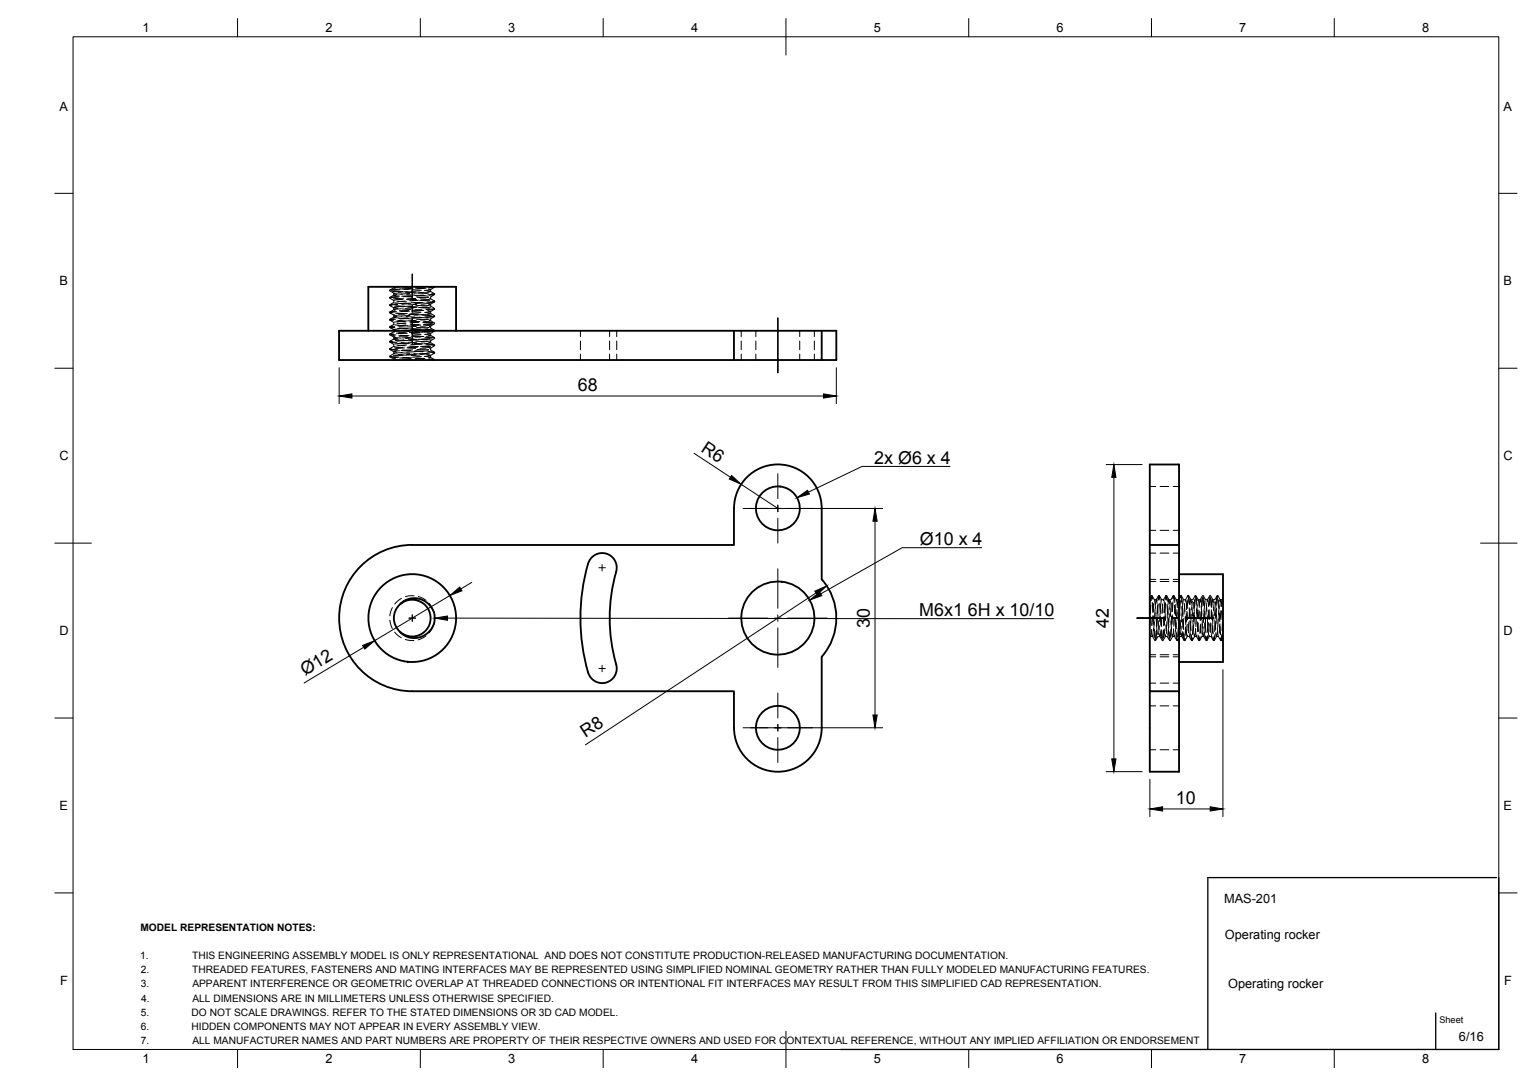
ISO-10303-21;
HEADER;
/* Generated by software containing ST-Developer
 * from STEP Tools, Inc. (www.steptools.com) 
 */

FILE_DESCRIPTION(
/* description */ ('Independent manual two-gate roller-track escapement for nominal30mm d
iameter20mm wide feed rollers. Opposed gates are driven by native capt
ured pin-slot loops with positive curved-slot travel stops at\X\B116de
g. Repeated gate/pin/washer/clip instances, adapted native common bear
ing families, full retaining lips and rotating polymer grip. External 
workpieces, gravity feeder/incline and mount anchors outside assembly.
 No powered-feed compatibility, impact, capacity, safety, force, wear 
or life rating.'),
/* implementation_level */ '2;1');

FILE_NAME(
/* name */ 'Operating rocker.step',
/* time_stamp */ '2026-11-08T18:43:23-08:00',
/* author */ (''),
/* organization */ (''),
/* preprocessor_version */ 'ST-DEVELOPER v20.2',
/* originating_system */ 'Autodesk Translation Framework v15.17.0.0',
/* authorisation */ '');

FILE_SCHEMA (('AUTOMOTIVE_DESIGN { 1 0 10303 214 3 1 1 }'));
ENDSEC;

DATA;
#10=MECHANICAL_DESIGN_GEOMETRIC_PRESENTATION_REPRESENTATION('',(#457),#19863);
#121=B_SPLINE_SURFACE_WITH_KNOTS('',3,3,((#14592,#14593,#14594,#14595,#14596,
#14597,#14598,#14599,#14600,#14601,#14602,#14603,#14604,#14605,#14606,#14607,
#14608,#14609,#14610,#14611,#14612,#14613,#14614,#14615,#14616,#14617,#14618,
#14619,#14620,#14621,#14622,#14623,#14624,#14625,#14626,#14627,#14628,#14629,
#14630,#14631,#14632,#14633,#14634,#14635,#14636,#14637,#14638,#14639,#14640,
#14641,#14642,#14643,#14644,#14645,#14646,#14647,#14648,#14649,#14650,#14651,
#14652,#14653,#14654,#14655,#14656,#14657,#14658,#14659),(#14660,#14661,
#14662,#14663,#14664,#14665,#14666,#14667,#14668,#14669,#14670,#14671,#14672,
#14673,#14674,#14675,#14676,#14677,#14678,#14679,#14680,#14681,#14682,#14683,
#14684,#14685,#14686,#14687,#14688,#14689,#14690,#14691,#14692,#14693,#14694,
#14695,#14696,#14697,#14698,#14699,#14700,#14701,#14702,#14703,#14704,#14705,
#14706,#14707,#14708,#14709,#14710,#14711,#14712,#14713,#14714,#14715,#14716,
#14717,#14718,#14719,#14720,#14721,#14722,#14723,#14724,#14725,#14726,#14727),
(#14728,#14729,#14730,#14731,#14732,#14733,#14734,#14735,#14736,#14737,
#14738,#14739,#14740,#14741,#14742,#14743,#14744,#14745,#14746,#14747,#14748,
#14749,#14750,#14751,#14752,#14753,#14754,#14755,#14756,#14757,#14758,#14759,
#14760,#14761,#14762,#14763,#14764,#14765,#14766,#14767,#14768,#14769,#14770,
#14771,#14772,#14773,#14774,#14775,#14776,#14777,#14778,#14779,#14780,#14781,
#14782,#14783,#14784,#14785,#14786,#14787,#14788,#14789,#14790,#14791,#14792,
#14793,#14794,#14795),(#14796,#14797,#14798,#14799,#14800,#14801,#14802,
#14803,#14804,#14805,#14806,#14807,#14808,#14809,#14810,#14811,#14812,#14813,
#14814,#14815,#14816,#14817,#14818,#14819,#14820,#14821,#14822,#14823,#14824,
#14825,#14826,#14827,#14828,#14829,#14830,#14831,#14832,#14833,#14834,#14835,
#14836,#14837,#14838,#14839,#14840,#14841,#14842,#14843,#14844,#14845,#14846,
#14847,#14848,#14849,#14850,#14851,#14852,#14853,#14854,#14855,#14856,#14857,
#14858,#14859,#14860,#14861,#14862,#14863)),.UNSPECIFIED.,.F.,.F.,.F.,(4,
4),(4,1,1,1,1,1,1,1,1,1,1,1,1,1,1,1,1,1,1,1,1,1,1,1,1,1,1,1,1,1,1,1,1,1,
1,1,1,1,1,1,1,1,1,1,1,1,1,1,1,1,1,1,1,1,1,1,1,1,1,1,1,1,1,1,1,4),(0.,0.0642013499338864),
(11.8589888623078,12.8566626771512,13.8543364919947,14.8520103068381,15.8496841216816,
16.8473579365251,17.8450317513685,18.842705566212,19.8403793810554,20.8380531958989,
21.8357270107423,22.8334008255858,23.8310746404292,24.8287484552727,25.8264222701161,
26.8240960849596,27.821769899803,28.8194437146465,29.8171175294899,30.8147913443334,
31.8124651591768,32.8101389740203,33.8078127888637,34.8054866037072,35.8031604185506,
36.8008342333941,37.7985080482375,38.796181863081,39.7938556779244,40.7915294927679,
41.7892033076113,42.7868771224548,43.7845509372982,44.7822247521417,45.7798985669851,
46.7775723818286,47.775246196672,48.7729200115155,49.7705938263589,50.7682676412024,
51.7659414560458,52.7636152708893,53.7612890857327,54.7589629005762,55.7566367154196,
56.7543105302631,57.7519843451065,58.74965815995,59.7473319747934,60.7450057896369,
61.7426796044803,62.7403534193238,63.7380272341672,64.7357010490107,65.7333748638542,
66.7310486786976,67.728722493541,68.7263963083845,69.7240701232279,70.7217439380714,
71.7194177529149,72.7170915677583,73.7147653826018,74.7124391974452,75.7101130122887,
76.7077868271321),.UNSPECIFIED.);
#122=B_SPLINE_SURFACE_WITH_KNOTS('',3,3,((#15080,#15081,#15082,#15083,#15084,
#15085,#15086,#15087,#15088,#15089,#15090,#15091,#15092,#15093,#15094,#15095,
#15096,#15097,#15098,#15099,#15100,#15101,#15102,#15103,#15104,#15105,#15106,
#15107,#15108,#15109,#15110,#15111,#15112,#15113,#15114,#15115,#15116,#15117,
#15118,#15119,#15120,#15121,#15122,#15123,#15124,#15125,#15126,#15127,#15128,
#15129,#15130,#15131,#15132,#15133,#15134,#15135,#15136,#15137,#15138,#15139,
#15140,#15141,#15142,#15143,#15144,#15145,#15146,#15147),(#15148,#15149,
#15150,#15151,#15152,#15153,#15154,#15155,#15156,#15157,#15158,#15159,#15160,
#15161,#15162,#15163,#15164,#15165,#15166,#15167,#15168,#15169,#15170,#15171,
#15172,#15173,#15174,#15175,#15176,#15177,#15178,#15179,#15180,#15181,#15182,
#15183,#15184,#15185,#15186,#15187,#15188,#15189,#15190,#15191,#15192,#15193,
#15194,#15195,#15196,#15197,#15198,#15199,#15200,#15201,#15202,#15203,#15204,
#15205,#15206,#15207,#15208,#15209,#15210,#15211,#15212,#15213,#15214,#15215),
(#15216,#15217,#15218,#15219,#15220,#15221,#15222,#15223,#15224,#15225,
#15226,#15227,#15228,#15229,#15230,#15231,#15232,#15233,#15234,#15235,#15236,
#15237,#15238,#15239,#15240,#15241,#15242,#15243,#15244,#15245,#15246,#15247,
#15248,#15249,#15250,#15251,#15252,#15253,#15254,#15255,#15256,#15257,#15258,
#15259,#15260,#15261,#15262,#15263,#15264,#15265,#15266,#15267,#15268,#15269,
#15270,#15271,#15272,#15273,#15274,#15275,#15276,#15277,#15278,#15279,#15280,
#15281,#15282,#15283),(#15284,#15285,#15286,#15287,#15288,#15289,#15290,
#15291,#15292,#15293,#15294,#15295,#15296,#15297,#15298,#15299,#15300,#15301,
#15302,#15303,#15304,#15305,#15306,#15307,#15308,#15309,#15310,#15311,#15312,
#15313,#15314,#15315,#15316,#15317,#15318,#15319,#15320,#15321,#15322,#15323,
#15324,#15325,#15326,#15327,#15328,#15329,#15330,#15331,#15332,#15333,#15334,
#15335,#15336,#15337,#15338,#15339,#15340,#15341,#15342,#15343,#15344,#15345,
#15346,#15347,#15348,#15349,#15350,#15351)),.UNSPECIFIED.,.F.,.F.,.F.,(4,
4),(4,1,1,1,1,1,1,1,1,1,1,1,1,1,1,1,1,1,1,1,1,1,1,1,1,1,1,1,1,1,1,1,1,1,
1,1,1,1,1,1,1,1,1,1,1,1,1,1,1,1,1,1,1,1,1,1,1,1,1,1,1,1,1,1,1,4),(0.,0.0642013499338864),
(14.3984001269718,15.3960739418153,16.3937477566587,17.3914215715022,18.3890953863456,
19.3867692011891,20.3844430160325,21.382116830876,22.3797906457194,23.3774644605629,
24.3751382754063,25.3728120902498,26.3704859050932,27.3681597199367,28.3658335347801,
29.3635073496236,30.361181164467,31.3588549793105,32.3565287941539,33.3542026089974,
34.3518764238408,35.3495502386843,36.3472240535278,37.3448978683712,38.3425716832147,
39.3402454980581,40.3379193129016,41.335593127745,42.3332669425885,43.3309407574319,
44.3286145722754,45.3262883871188,46.3239622019623,47.3216360168057,48.3193098316492,
49.3169836464926,50.3146574613361,51.3123312761795,52.310005091023,53.3076789058664,
54.3053527207099,55.3030265355533,56.3007003503968,57.2983741652402,58.2960479800837,
59.2937217949271,60.2913956097706,61.289069424614,62.2867432394575,63.2844170543009,
64.2820908691444,65.2797646839878,66.2774384988313,67.2751123136747,68.2727861285182,
69.2704599433616,70.2681337582051,71.2658075730485,72.263481387892,73.2611552027354,
74.2588290175789,75.2565028324223,76.2541766472658,77.2518504621092,78.2495242769527,
79.2471980917962),.UNSPECIFIED.);
#269=B_SPLINE_CURVE_WITH_KNOTS('',3,(#13855,#13856,#13857,#13858),
 .UNSPECIFIED.,.F.,.F.,(4,4),(64.141416212773,64.8487979648243),
 .UNSPECIFIED.);
#270=B_SPLINE_CURVE_WITH_KNOTS('',3,(#13861,#13862,#13863,#13864,#13865,
#13866,#13867,#13868,#13869,#13870),.UNSPECIFIED.,.F.,.F.,(4,3,3,4),(-62.8318530717959,
-61.855776520294,-60.8581027054505,-60.3976421702574),.UNSPECIFIED.);
#271=B_SPLINE_CURVE_WITH_KNOTS('',3,(#13875,#13876,#13877,#13878,#13879,
#13880,#13881,#13882,#13883,#13884,#13885,#13886,#13887,#13888,#13889,#13890,
#13891,#13892,#13893,#13894,#13895,#13896,#13897,#13898,#13899),
 .UNSPECIFIED.,.F.,.F.,(4,3,3,3,3,3,3,3,4),(57.8582309055934,57.8650812609202,
58.8627550757636,59.8604288906071,60.8581027054505,61.855776520294,62.8534503351374,
63.8511241499809,64.141416212773),.UNSPECIFIED.);
#272=B_SPLINE_CURVE_WITH_KNOTS('',3,(#13900,#13901,#13902,#13903,#13904,
#13905,#13906,#13907,#13908,#13909,#13910,#13911,#13912,#13913,#13914,#13915,
#13916,#13917,#13918,#13919,#13920,#13921),.UNSPECIFIED.,.F.,.F.,(4,3,3,
3,3,3,3,4),(-60.3976421702574,-59.8604288906071,-58.8627550757636,-57.8650812609202,
-56.8674074460767,-55.8697336312333,-54.8720598163898,-54.1144568630778),
 .UNSPECIFIED.);
#273=B_SPLINE_CURVE_WITH_KNOTS('',3,(#13926,#13927,#13928,#13929,#13930,
#13931,#13932,#13933,#13934,#13935,#13936,#13937,#13938,#13939,#13940,#13941,
#13942,#13943,#13944,#13945,#13946,#13947),.UNSPECIFIED.,.F.,.F.,(4,3,3,
3,3,3,3,4),(51.5750455984138,51.8790383718595,52.8767121867029,53.8743860015464,
54.8720598163898,55.8697336312333,56.8674074460767,57.8582309055934),
 .UNSPECIFIED.);
#274=B_SPLINE_CURVE_WITH_KNOTS('',3,(#13948,#13949,#13950,#13951,#13952,
#13953,#13954,#13955,#13956,#13957,#13958,#13959,#13960,#13961,#13962,#13963,
#13964,#13965,#13966,#13967,#13968,#13969,#13970,#13971,#13972),
 .UNSPECIFIED.,.F.,.F.,(4,3,3,3,3,3,3,3,4),(-54.1144568630778,-53.8743860015464,
-52.8767121867029,-51.8790383718595,-50.881364557016,-49.8836907421725,
-48.8860169273291,-47.8883431124856,-47.8312715558982),.UNSPECIFIED.);
#275=B_SPLINE_CURVE_WITH_KNOTS('',3,(#13977,#13978,#13979,#13980,#13981,
#13982,#13983,#13984,#13985,#13986,#13987,#13988,#13989,#13990,#13991,#13992,
#13993,#13994,#13995,#13996,#13997,#13998),.UNSPECIFIED.,.F.,.F.,(4,3,3,
3,3,3,3,4),(45.2918602912342,45.8929954827987,46.8906692976422,47.8883431124856,
48.8860169273291,49.8836907421725,50.881364557016,51.5750455984138),
 .UNSPECIFIED.);
#276=B_SPLINE_CURVE_WITH_KNOTS('',3,(#13999,#14000,#14001,#14002,#14003,
#14004,#14005,#14006,#14007,#14008,#14009,#14010,#14011,#14012,#14013,#14014,
#14015,#14016,#14017,#14018,#14019,#14020),.UNSPECIFIED.,.F.,.F.,(4,3,3,
3,3,3,3,4),(-47.8312715558982,-46.8906692976422,-45.8929954827987,-44.8953216679553,
-43.8976478531118,-42.8999740382684,-41.9023002234249,-41.5480862487187),
 .UNSPECIFIED.);
#277=B_SPLINE_CURVE_WITH_KNOTS('',3,(#14025,#14026,#14027,#14028,#14029,
#14030,#14031,#14032,#14033,#14034,#14035,#14036,#14037,#14038,#14039,#14040,
#14041,#14042,#14043,#14044,#14045,#14046),.UNSPECIFIED.,.F.,.F.,(4,3,3,
3,3,3,3,4),(39.0086749840546,39.906952593738,40.9046264085815,41.9023002234249,
42.8999740382684,43.8976478531118,44.8953216679553,45.2918602912342),
 .UNSPECIFIED.);
#278=B_SPLINE_CURVE_WITH_KNOTS('',3,(#14047,#14048,#14049,#14050,#14051,
#14052,#14053,#14054,#14055,#14056,#14057,#14058,#14059,#14060,#14061,#14062,
#14063,#14064,#14065,#14066,#14067,#14068),.UNSPECIFIED.,.F.,.F.,(4,3,3,
3,3,3,3,4),(-41.5480862487187,-40.9046264085815,-39.906952593738,-38.9092787788946,
-37.9116049640511,-36.9139311492077,-35.9162573343642,-35.2649009415391),
 .UNSPECIFIED.);
#279=B_SPLINE_CURVE_WITH_KNOTS('',3,(#14073,#14074,#14075,#14076,#14077,
#14078,#14079,#14080,#14081,#14082,#14083,#14084,#14085,#14086,#14087,#14088,
#14089,#14090,#14091,#14092,#14093,#14094,#14095,#14096,#14097),
 .UNSPECIFIED.,.F.,.F.,(4,3,3,3,3,3,3,3,4),(32.725489676875,32.9232358898339,
33.9209097046773,34.9185835195208,35.9162573343642,36.9139311492077,37.9116049640511,
38.9092787788946,39.0086749840546),.UNSPECIFIED.);
#280=B_SPLINE_CURVE_WITH_KNOTS('',3,(#14098,#14099,#14100,#14101,#14102,
#14103,#14104,#14105,#14106,#14107,#14108,#14109,#14110,#14111,#14112,#14113,
#14114,#14115,#14116,#14117,#14118,#14119),.UNSPECIFIED.,.F.,.F.,(4,3,3,
3,3,3,3,4),(-35.2649009415391,-34.9185835195208,-33.9209097046773,-32.9232358898339,
-31.9255620749904,-30.927888260147,-29.9302144453035,-28.9817156343595),
 .UNSPECIFIED.);
#281=B_SPLINE_CURVE_WITH_KNOTS('',3,(#14124,#14125,#14126,#14127,#14128,
#14129,#14130,#14131,#14132,#14133,#14134,#14135,#14136,#14137,#14138,#14139,
#14140,#14141,#14142,#14143,#14144,#14145),.UNSPECIFIED.,.F.,.F.,(4,3,3,
3,3,3,3,4),(26.4423043696954,26.9371930007732,27.9348668156166,28.9325406304601,
29.9302144453035,30.927888260147,31.9255620749904,32.725489676875),
 .UNSPECIFIED.);
#282=B_SPLINE_CURVE_WITH_KNOTS('',3,(#14146,#14147,#14148,#14149,#14150,
#14151,#14152,#14153,#14154,#14155,#14156,#14157,#14158,#14159,#14160,#14161,
#14162,#14163,#14164,#14165,#14166,#14167,#14168,#14169,#14170),
 .UNSPECIFIED.,.F.,.F.,(4,3,3,3,3,3,3,3,4),(-28.9817156343595,-28.9325406304601,
-27.9348668156166,-26.9371930007732,-25.9395191859297,-24.9418453710863,
-23.9441715562428,-22.9464977413994,-22.6985303271799),.UNSPECIFIED.);
#283=B_SPLINE_CURVE_WITH_KNOTS('',3,(#14175,#14176,#14177,#14178,#14179,
#14180,#14181,#14182,#14183,#14184,#14185,#14186,#14187,#14188,#14189,#14190,
#14191,#14192,#14193,#14194,#14195,#14196),.UNSPECIFIED.,.F.,.F.,(4,3,3,
3,3,3,3,4),(20.1591190625158,20.9511501117125,21.9488239265559,22.9464977413994,
23.9441715562428,24.9418453710863,25.9395191859297,26.4423043696954),
 .UNSPECIFIED.);
#284=B_SPLINE_CURVE_WITH_KNOTS('',3,(#14197,#14198,#14199,#14200,#14201,
#14202,#14203,#14204,#14205,#14206,#14207,#14208,#14209,#14210,#14211,#14212,
#14213,#14214,#14215,#14216,#14217,#14218),.UNSPECIFIED.,.F.,.F.,(4,3,3,
3,3,3,3,4),(-22.6985303271799,-21.9488239265559,-20.9511501117125,-19.953476296869,
-18.9558024820256,-17.9581286671821,-16.9604548523387,-16.4153450200003),
 .UNSPECIFIED.);
#285=B_SPLINE_CURVE_WITH_KNOTS('',3,(#14223,#14224,#14225,#14226,#14227,
#14228,#14229,#14230,#14231,#14232,#14233,#14234,#14235,#14236,#14237,#14238,
#14239,#14240,#14241,#14242,#14243,#14244,#14245,#14246,#14247),
 .UNSPECIFIED.,.F.,.F.,(4,3,3,3,3,3,3,3,4),(13.8759337553362,13.9674334078083,
14.9651072226518,15.9627810374952,16.9604548523387,17.9581286671821,18.9558024820256,
19.953476296869,20.1591190625158),.UNSPECIFIED.);
#286=B_SPLINE_CURVE_WITH_KNOTS('',3,(#14248,#14249,#14250,#14251,#14252,
#14253,#14254,#14255,#14256,#14257,#14258,#14259,#14260,#14261,#14262,#14263,
#14264,#14265,#14266,#14267,#14268,#14269),.UNSPECIFIED.,.F.,.F.,(4,3,3,
3,3,3,3,4),(-16.4153450200003,-15.9627810374952,-14.9651072226518,-13.9674334078083,
-12.9697595929649,-11.9720857781214,-10.974411963278,-10.1321597128207),
 .UNSPECIFIED.);
#287=B_SPLINE_CURVE_WITH_KNOTS('',3,(#14275,#14276,#14277,#14278,#14279,
#14280,#14281,#14282,#14283,#14284,#14285,#14286,#14287),.UNSPECIFIED.,
 .F.,.F.,(4,3,3,3,4),(-3.84897440564113,-2.99302144453035,-1.9953476296869,
-0.997673814843452,0.),.UNSPECIFIED.);
#288=B_SPLINE_CURVE_WITH_KNOTS('',3,(#14290,#14291,#14292,#14293,#14294,
#14295,#14296,#14297,#14298,#14299,#14300,#14301,#14302,#14303,#14304,#14305,
#14306,#14307,#14308),.UNSPECIFIED.,.F.,.F.,(4,3,3,3,3,3,4),(2.01694489302847,
2.99302144453035,3.9906952593738,4.98836907421726,5.98604288906071,6.98371670390416,
7.59274844815664),.UNSPECIFIED.);
#289=B_SPLINE_CURVE_WITH_KNOTS('',3,(#14314,#14315,#14316,#14317,#14318,
#14319,#14320,#14321),.UNSPECIFIED.,.F.,.F.,(4,1,1,1,1,4),(72.2566310325652,
72.7170915677583,73.7147653826018,74.7124391974452,75.7101130122887,76.7077868271321),
 .UNSPECIFIED.);
#290=B_SPLINE_CURVE_WITH_KNOTS('',3,(#14324,#14325,#14326,#14327,#14328,
#14329,#14330,#14331,#14332),.UNSPECIFIED.,.F.,.F.,(4,1,1,1,1,1,4),(72.2566310325652,
72.263481387892,73.2611552027354,74.2588290175789,75.2565028324223,76.2541766472658,
77.2302531987677),.UNSPECIFIED.);
#291=B_SPLINE_CURVE_WITH_KNOTS('',3,(#14337,#14338,#14339,#14340,#14341,
#14342,#14343,#14344,#14345,#14346),.UNSPECIFIED.,.F.,.F.,(4,1,1,1,1,1,
1,4),(65.9734457253856,66.7310486786976,67.728722493541,68.7263963083845,
69.7240701232279,70.7217439380714,71.7194177529149,72.2566310325652),
 .UNSPECIFIED.);
#292=B_SPLINE_CURVE_WITH_KNOTS('',3,(#14347,#14348,#14349,#14350,#14351,
#14352,#14353,#14354,#14355,#14356),.UNSPECIFIED.,.F.,.F.,(4,1,1,1,1,1,
1,4),(65.9734457253856,66.2774384988313,67.2751123136747,68.2727861285182,
69.2704599433616,70.2681337582051,71.2658075730485,72.2566310325652),
 .UNSPECIFIED.);
#293=B_SPLINE_CURVE_WITH_KNOTS('',3,(#14361,#14362,#14363,#14364,#14365,
#14366,#14367,#14368,#14369,#14370,#14371),.UNSPECIFIED.,.F.,.F.,(4,1,1,
1,1,1,1,1,4),(59.6902604182061,59.7473319747934,60.7450057896369,61.7426796044803,
62.7403534193238,63.7380272341672,64.7357010490107,65.7333748638542,65.9734457253856),
 .UNSPECIFIED.);
#294=B_SPLINE_CURVE_WITH_KNOTS('',3,(#14372,#14373,#14374,#14375,#14376,
#14377,#14378,#14379,#14380,#14381),.UNSPECIFIED.,.F.,.F.,(4,1,1,1,1,1,
1,4),(59.6902604182061,60.2913956097706,61.289069424614,62.2867432394575,
63.2844170543009,64.2820908691444,65.2797646839878,65.9734457253856),
 .UNSPECIFIED.);
#295=B_SPLINE_CURVE_WITH_KNOTS('',3,(#14386,#14387,#14388,#14389,#14390,
#14391,#14392,#14393,#14394,#14395),.UNSPECIFIED.,.F.,.F.,(4,1,1,1,1,1,
1,4),(53.4070751110265,53.7612890857327,54.7589629005762,55.7566367154196,
56.7543105302631,57.7519843451065,58.74965815995,59.6902604182061),
 .UNSPECIFIED.);
#296=B_SPLINE_CURVE_WITH_KNOTS('',3,(#14396,#14397,#14398,#14399,#14400,
#14401,#14402,#14403,#14404,#14405),.UNSPECIFIED.,.F.,.F.,(4,1,1,1,1,1,
1,4),(53.4070751110265,54.3053527207099,55.3030265355533,56.3007003503968,
57.2983741652402,58.2960479800837,59.2937217949271,59.6902604182061),
 .UNSPECIFIED.);
#297=B_SPLINE_CURVE_WITH_KNOTS('',3,(#14410,#14411,#14412,#14413,#14414,
#14415,#14416,#14417,#14418,#14419),.UNSPECIFIED.,.F.,.F.,(4,1,1,1,1,1,
1,4),(47.1238898038469,47.775246196672,48.7729200115155,49.7705938263589,
50.7682676412024,51.7659414560458,52.7636152708893,53.4070751110265),
 .UNSPECIFIED.);
#298=B_SPLINE_CURVE_WITH_KNOTS('',3,(#14420,#14421,#14422,#14423,#14424,
#14425,#14426,#14427,#14428,#14429,#14430),.UNSPECIFIED.,.F.,.F.,(4,1,1,
1,1,1,1,1,4),(47.1238898038469,47.3216360168057,48.3193098316492,49.3169836464926,
50.3146574613361,51.3123312761795,52.310005091023,53.3076789058664,53.4070751110265),
 .UNSPECIFIED.);
#299=B_SPLINE_CURVE_WITH_KNOTS('',3,(#14435,#14436,#14437,#14438,#14439,
#14440,#14441,#14442,#14443,#14444),.UNSPECIFIED.,.F.,.F.,(4,1,1,1,1,1,
1,4),(40.8407044966673,41.7892033076113,42.7868771224548,43.7845509372982,
44.7822247521417,45.7798985669851,46.7775723818286,47.1238898038469),
 .UNSPECIFIED.);
#300=B_SPLINE_CURVE_WITH_KNOTS('',3,(#14445,#14446,#14447,#14448,#14449,
#14450,#14451,#14452,#14453,#14454),.UNSPECIFIED.,.F.,.F.,(4,1,1,1,1,1,
1,4),(40.8407044966673,41.335593127745,42.3332669425885,43.3309407574319,
44.3286145722754,45.3262883871188,46.3239622019623,47.1238898038469),
 .UNSPECIFIED.);
#301=B_SPLINE_CURVE_WITH_KNOTS('',3,(#14459,#14460,#14461,#14462,#14463,
#14464,#14465,#14466,#14467,#14468,#14469),.UNSPECIFIED.,.F.,.F.,(4,1,1,
1,1,1,1,1,4),(34.5575191894877,34.8054866037072,35.8031604185506,36.8008342333941,
37.7985080482375,38.796181863081,39.7938556779244,40.7915294927679,40.8407044966673),
 .UNSPECIFIED.);
#302=B_SPLINE_CURVE_WITH_KNOTS('',3,(#14470,#14471,#14472,#14473,#14474,
#14475,#14476,#14477,#14478,#14479),.UNSPECIFIED.,.F.,.F.,(4,1,1,1,1,1,
1,4),(34.5575191894877,35.3495502386843,36.3472240535278,37.3448978683712,
38.3425716832147,39.3402454980581,40.3379193129016,40.8407044966673),
 .UNSPECIFIED.);
#303=B_SPLINE_CURVE_WITH_KNOTS('',3,(#14484,#14485,#14486,#14487,#14488,
#14489,#14490,#14491,#14492,#14493),.UNSPECIFIED.,.F.,.F.,(4,1,1,1,1,1,
1,4),(28.2743338823081,28.8194437146465,29.8171175294899,30.8147913443334,
31.8124651591768,32.8101389740203,33.8078127888637,34.5575191894877),
 .UNSPECIFIED.);
#304=B_SPLINE_CURVE_WITH_KNOTS('',3,(#14494,#14495,#14496,#14497,#14498,
#14499,#14500,#14501,#14502,#14503,#14504),.UNSPECIFIED.,.F.,.F.,(4,1,1,
1,1,1,1,1,4),(28.2743338823081,28.3658335347801,29.3635073496236,30.361181164467,
31.3588549793105,32.3565287941539,33.3542026089974,34.3518764238408,34.5575191894877),
 .UNSPECIFIED.);
#305=B_SPLINE_CURVE_WITH_KNOTS('',3,(#14509,#14510,#14511,#14512,#14513,
#14514,#14515,#14516,#14517,#14518),.UNSPECIFIED.,.F.,.F.,(4,1,1,1,1,1,
1,4),(21.9911485751285,22.8334008255858,23.8310746404292,24.8287484552727,
25.8264222701161,26.8240960849596,27.821769899803,28.2743338823081),
 .UNSPECIFIED.);
#306=B_SPLINE_CURVE_WITH_KNOTS('',3,(#14519,#14520,#14521,#14522,#14523,
#14524,#14525,#14526,#14527,#14528),.UNSPECIFIED.,.F.,.F.,(4,1,1,1,1,1,
1,4),(21.9911485751285,22.3797906457194,23.3774644605629,24.3751382754063,
25.3728120902498,26.3704859050932,27.3681597199367,28.2743338823081),
 .UNSPECIFIED.);
#307=B_SPLINE_CURVE_WITH_KNOTS('',3,(#14534,#14535,#14536,#14537,#14538),
 .UNSPECIFIED.,.F.,.F.,(4,1,4),(14.3984001269718,15.3960739418153,15.7079632679489),
 .UNSPECIFIED.);
#308=B_SPLINE_CURVE_WITH_KNOTS('',3,(#14541,#14542,#14543,#14544,#14545),
 .UNSPECIFIED.,.F.,.F.,(4,1,4),(13.8759337553362,14.8520103068381,15.7079632679489),
 .UNSPECIFIED.);
#309=B_SPLINE_CURVE_WITH_KNOTS('',3,(#14571,#14572,#14573,#14574,#14575,
#14576,#14577,#14578,#14579,#14580,#14581),.UNSPECIFIED.,.F.,.F.,(4,1,1,
1,1,1,1,1,4),(15.7079632679489,15.8496841216816,16.8473579365251,17.8450317513685,
18.842705566212,19.8403793810554,20.8380531958989,21.8357270107423,21.9911485751285),
 .UNSPECIFIED.);
#310=B_SPLINE_CURVE_WITH_KNOTS('',3,(#14582,#14583,#14584,#14585,#14586,
#14587,#14588,#14589,#14590,#14591),.UNSPECIFIED.,.F.,.F.,(4,1,1,1,1,1,
1,4),(15.7079632679489,16.3937477566587,17.3914215715022,18.3890953863456,
19.3867692011891,20.3844430160325,21.382116830876,21.9911485751285),
 .UNSPECIFIED.);
#311=B_SPLINE_CURVE_WITH_KNOTS('',3,(#14864,#14865,#14866,#14867,#14868,
#14869,#14870,#14871,#14872,#14873,#14874,#14875,#14876,#14877,#14878,#14879,
#14880,#14881,#14882,#14883,#14884,#14885,#14886,#14887,#14888,#14889,#14890,
#14891,#14892,#14893,#14894,#14895,#14896,#14897,#14898,#14899,#14900,#14901,
#14902,#14903,#14904,#14905,#14906,#14907,#14908,#14909,#14910,#14911,#14912,
#14913,#14914,#14915,#14916,#14917,#14918,#14919,#14920,#14921,#14922,#14923,
#14924,#14925,#14926,#14927,#14928,#14929,#14930,#14931,#14932,#14933,#14934,
#14935,#14936,#14937,#14938,#14939,#14940,#14941,#14942,#14943,#14944,#14945,
#14946,#14947,#14948,#14949,#14950,#14951,#14952,#14953,#14954,#14955,#14956,
#14957),.UNSPECIFIED.,.F.,.F.,(4,3,3,3,3,3,3,3,3,3,3,3,3,3,3,3,3,3,3,3,
3,3,3,3,3,3,3,3,3,3,3,4),(0.,0.0297266436256191,0.060112679207304,0.0895302342422888,
0.115270594897901,0.120663503251604,0.150426428066333,0.180024192439473,
0.208881424201401,0.221328323689936,0.230189025923113,0.234057622905472,
0.262601272727233,0.290514012411483,0.295453119487182,0.324405121619328,
0.334115029800546,0.339546867385313,0.343311613769743,0.371402114253626,
0.399548690384148,0.427297276293485,0.438085418679347,0.44385539363774,
0.448937718500496,0.477641070286612,0.499168584126198,0.508042229411102,
0.513343363411791,0.539241448194656,0.563751125644958,0.56924861039943),
 .UNSPECIFIED.);
#312=B_SPLINE_CURVE_WITH_KNOTS('',3,(#14958,#14959,#14960,#14961,#14962,
#14963,#14964,#14965,#14966,#14967,#14968,#14969,#14970,#14971,#14972,#14973,
#14974,#14975,#14976,#14977,#14978,#14979,#14980,#14981,#14982,#14983,#14984,
#14985,#14986,#14987,#14988,#14989,#14990,#14991,#14992,#14993,#14994,#14995,
#14996,#14997,#14998,#14999,#15000,#15001,#15002,#15003,#15004,#15005,#15006,
#15007,#15008,#15009,#15010,#15011,#15012,#15013,#15014,#15015,#15016,#15017,
#15018,#15019,#15020,#15021,#15022,#15023,#15024,#15025,#15026,#15027,#15028,
#15029,#15030,#15031,#15032,#15033,#15034,#15035,#15036,#15037,#15038,#15039,
#15040,#15041,#15042,#15043,#15044,#15045,#15046,#15047,#15048,#15049,#15050,
#15051,#15052,#15053,#15054),.UNSPECIFIED.,.F.,.F.,(4,3,3,3,3,3,3,3,3,3,
3,3,3,3,3,3,3,3,3,3,3,3,3,3,3,3,3,3,3,3,3,3,4),(0.,0.0253663834374841,0.0514041120650232,
0.0783366031747472,0.0901195680352514,0.0965544176388419,0.102698656155734,
0.130005061278407,0.157761496023994,0.185037132253699,0.195822334387975,
0.20220621696723,0.20645540248052,0.235058614057351,0.263563013331617,0.266864040942815,
0.294770641765994,0.305810449331027,0.3111858125117,0.31568945545677,0.343780872272608,
0.372913770005713,0.40236688452419,0.41382997653101,0.422924087167126,0.42812442164653,
0.458189344870008,0.483694943608004,0.492094089615772,0.498168184514284,
0.529189962168139,0.560211739821994,0.566847306048124),.UNSPECIFIED.);
#313=B_SPLINE_CURVE_WITH_KNOTS('',3,(#15055,#15056,#15057,#15058,#15059,
#15060,#15061,#15062,#15063,#15064,#15065,#15066,#15067,#15068,#15069,#15070,
#15071,#15072,#15073,#15074,#15075,#15076,#15077,#15078,#15079),
 .UNSPECIFIED.,.F.,.F.,(4,3,3,3,3,3,3,3,4),(-10.1321597128207,-9.97673814843451,
-8.97906433359106,-7.98139051874761,-6.98371670390416,-5.9860428890607,
-4.98836907421726,-3.99069525937381,-3.84897440564113),.UNSPECIFIED.);
#314=B_SPLINE_CURVE_WITH_KNOTS('',3,(#15352,#15353,#15354,#15355,#15356,
#15357,#15358,#15359,#15360,#15361,#15362,#15363,#15364,#15365,#15366,#15367,
#15368,#15369,#15370,#15371,#15372,#15373,#15374,#15375,#15376,#15377,#15378,
#15379,#15380,#15381,#15382,#15383,#15384,#15385,#15386,#15387,#15388,#15389,
#15390,#15391,#15392,#15393,#15394,#15395,#15396,#15397,#15398,#15399,#15400,
#15401,#15402,#15403,#15404,#15405,#15406,#15407,#15408,#15409,#15410,#15411,
#15412,#15413,#15414,#15415,#15416,#15417,#15418,#15419,#15420,#15421,#15422,
#15423,#15424,#15425,#15426,#15427,#15428,#15429,#15430,#15431,#15432,#15433,
#15434,#15435,#15436,#15437,#15438,#15439,#15440,#15441,#15442,#15443,#15444,
#15445,#15446,#15447,#15448),.UNSPECIFIED.,.F.,.F.,(4,3,3,3,3,3,3,3,3,3,
3,3,3,3,3,3,3,3,3,3,3,3,3,3,3,3,3,3,3,3,3,3,4),(0.,0.0253664359602338,0.0514042119244802,
0.0783366905517712,0.0901196499512111,0.0965544540618819,0.102698644967743,
0.130005086208347,0.157761538287333,0.185037163951202,0.195822342994834,
0.20220622673851,0.206455408544716,0.235058628439391,0.26356301086795,0.266864040942809,
0.29477061610912,0.305810395174784,0.311185261381901,0.315689367741021,
0.343780744986089,0.372913624523944,0.402366734593413,0.413829681327142,
0.422920909218603,0.428124127377988,0.458189039903474,0.483694714883097,
0.492093067075374,0.498168205826972,0.529189972824469,0.560211739821966,
0.566847306048091),.UNSPECIFIED.);
#315=B_SPLINE_CURVE_WITH_KNOTS('',3,(#15449,#15450,#15451,#15452,#15453,
#15454,#15455,#15456,#15457,#15458,#15459,#15460,#15461,#15462,#15463,#15464,
#15465,#15466,#15467,#15468,#15469,#15470),.UNSPECIFIED.,.F.,.F.,(4,3,3,
3,3,3,3,4),(7.59274844815664,7.98139051874761,8.97906433359106,9.97673814843451,
10.974411963278,11.9720857781214,12.9697595929649,13.8759337553362),
 .UNSPECIFIED.);
#316=B_SPLINE_CURVE_WITH_KNOTS('',3,(#15471,#15472,#15473,#15474,#15475,
#15476,#15477,#15478,#15479,#15480,#15481,#15482,#15483,#15484,#15485,#15486,
#15487,#15488,#15489,#15490,#15491,#15492,#15493,#15494,#15495,#15496,#15497,
#15498,#15499,#15500,#15501,#15502,#15503,#15504,#15505,#15506,#15507,#15508,
#15509,#15510,#15511,#15512,#15513,#15514,#15515,#15516,#15517,#15518,#15519,
#15520,#15521,#15522,#15523,#15524,#15525,#15526,#15527,#15528,#15529,#15530,
#15531,#15532,#15533,#15534,#15535,#15536,#15537,#15538,#15539,#15540,#15541,
#15542,#15543,#15544,#15545,#15546,#15547,#15548,#15549,#15550,#15551,#15552,
#15553,#15554,#15555,#15556,#15557,#15558,#15559,#15560,#15561,#15562,#15563,
#15564),.UNSPECIFIED.,.F.,.F.,(4,3,3,3,3,3,3,3,3,3,3,3,3,3,3,3,3,3,3,3,
3,3,3,3,3,3,3,3,3,3,3,4),(0.,0.0297266875030074,0.0601127445946389,0.0895302914562022,
0.11527064496007,0.120663513700728,0.150426438565439,0.180024190458537,
0.208881422715689,0.221328316071619,0.23018892405708,0.234057477327688,
0.262601114877733,0.290513844971786,0.295453119487145,0.32440512352943,
0.334115024654919,0.339546862874593,0.343311606495589,0.371402108073593,
0.399548683927862,0.427297259020053,0.438085377485613,0.443855354480411,
0.448937716391162,0.477641068704603,0.499168582939684,0.508042210823306,
0.513343356614935,0.539241415166652,0.563751125644927,0.569248610399403),
 .UNSPECIFIED.);
#419=SHAPE_REPRESENTATION_RELATIONSHIP('SRR','None',#19937,#438);
#438=ADVANCED_BREP_SHAPE_REPRESENTATION('',(#476),#19846);
#457=STYLED_ITEM('',(#20039),#476);
#476=MANIFOLD_SOLID_BREP('Body1',#6426);
#724=LINE('',#13853,#1189);
#725=LINE('',#13874,#1190);
#726=LINE('',#13925,#1191);
#727=LINE('',#13976,#1192);
#728=LINE('',#14024,#1193);
#729=LINE('',#14072,#1194);
#730=LINE('',#14123,#1195);
#731=LINE('',#14174,#1196);
#732=LINE('',#14222,#1197);
#733=LINE('',#14273,#1198);
#734=LINE('',#14312,#1199);
#735=LINE('',#14336,#1200);
#736=LINE('',#14360,#1201);
#737=LINE('',#14385,#1202);
#738=LINE('',#14409,#1203);
#739=LINE('',#14434,#1204);
#740=LINE('',#14458,#1205);
#741=LINE('',#14483,#1206);
#742=LINE('',#14508,#1207);
#743=LINE('',#14532,#1208);
#744=LINE('',#14551,#1209);
#745=LINE('',#14554,#1210);
#746=LINE('',#14559,#1211);
#747=LINE('',#14565,#1212);
#748=LINE('',#15573,#1213);
#749=LINE('',#15579,#1214);
#750=LINE('',#15585,#1215);
#751=LINE('',#15589,#1216);
#752=LINE('',#15594,#1217);
#753=LINE('',#15598,#1218);
#754=LINE('',#15602,#1219);
#755=LINE('',#15604,#1220);
#756=LINE('',#15608,#1221);
#757=LINE('',#15612,#1222);
#758=LINE('',#15616,#1223);
#759=LINE('',#15617,#1224);
#760=LINE('',#15620,#1225);
#761=LINE('',#15621,#1226);
#762=LINE('',#15624,#1227);
#763=LINE('',#15625,#1228);
#764=LINE('',#15628,#1229);
#765=LINE('',#15629,#1230);
#766=LINE('',#15632,#1231);
#767=LINE('',#15636,#1232);
#768=LINE('',#15640,#1233);
#769=LINE('',#15643,#1234);
#770=LINE('',#15644,#1235);
#771=LINE('',#15646,#1236);
#772=LINE('',#15648,#1237);
#773=LINE('',#15650,#1238);
#1189=VECTOR('',#7774,3.);
#1190=VECTOR('',#7779,3.);
#1191=VECTOR('',#7782,3.);
#1192=VECTOR('',#7785,3.);
#1193=VECTOR('',#7788,3.);
#1194=VECTOR('',#7791,3.);
#1195=VECTOR('',#7794,3.);
#1196=VECTOR('',#7797,3.);
#1197=VECTOR('',#7800,3.);
#1198=VECTOR('',#7803,3.);
#1199=VECTOR('',#7808,3.0735);
#1200=VECTOR('',#7813,3.0735);
#1201=VECTOR('',#7816,3.0735);
#1202=VECTOR('',#7819,3.0735);
#1203=VECTOR('',#7822,3.0735);
#1204=VECTOR('',#7825,3.0735);
#1205=VECTOR('',#7828,3.0735);
#1206=VECTOR('',#7831,3.0735);
#1207=VECTOR('',#7834,3.0735);
#1208=VECTOR('',#7837,3.0735);
#1209=VECTOR('',#7844,10.);
#1210=VECTOR('',#7847,10.);
#1211=VECTOR('',#7852,10.);
#1212=VECTOR('',#7859,10.);
#1213=VECTOR('',#7880,3.);
#1214=VECTOR('',#7887,3.);
#1215=VECTOR('',#7894,5.);
#1216=VECTOR('',#7899,6.);
#1217=VECTOR('',#7904,10.);
#1218=VECTOR('',#7907,10.);
#1219=VECTOR('',#7912,10.);
#1220=VECTOR('',#7913,10.);
#1221=VECTOR('',#7916,10.);
#1222=VECTOR('',#7919,10.);
#1223=VECTOR('',#7922,10.);
#1224=VECTOR('',#7923,10.);
#1225=VECTOR('',#7926,10.);
#1226=VECTOR('',#7927,10.);
#1227=VECTOR('',#7930,10.);
#1228=VECTOR('',#7931,10.);
#1229=VECTOR('',#7934,10.);
#1230=VECTOR('',#7935,10.);
#1231=VECTOR('',#7938,10.);
#1232=VECTOR('',#7941,10.);
#1233=VECTOR('',#7944,10.);
#1234=VECTOR('',#7949,10.);
#1235=VECTOR('',#7950,10.);
#1236=VECTOR('',#7953,10.);
#1237=VECTOR('',#7956,10.);
#1238=VECTOR('',#7959,10.);
#1500=CYLINDRICAL_SURFACE('',#6828,2.5175);
#1501=CYLINDRICAL_SURFACE('',#6830,2.5175);
#1502=CYLINDRICAL_SURFACE('',#6831,2.5175);
#1503=CYLINDRICAL_SURFACE('',#6832,2.5175);
#1504=CYLINDRICAL_SURFACE('',#6833,2.5175);
#1505=CYLINDRICAL_SURFACE('',#6834,2.5175);
#1506=CYLINDRICAL_SURFACE('',#6835,2.5175);
#1507=CYLINDRICAL_SURFACE('',#6836,2.5175);
#1508=CYLINDRICAL_SURFACE('',#6837,2.5175);
#1509=CYLINDRICAL_SURFACE('',#6838,2.5175);
#1510=CYLINDRICAL_SURFACE('',#6840,3.0735);
#1511=CYLINDRICAL_SURFACE('',#6842,3.0735);
#1512=CYLINDRICAL_SURFACE('',#6843,3.0735);
#1513=CYLINDRICAL_SURFACE('',#6844,3.0735);
#1514=CYLINDRICAL_SURFACE('',#6845,3.0735);
#1515=CYLINDRICAL_SURFACE('',#6846,3.0735);
#1516=CYLINDRICAL_SURFACE('',#6847,3.0735);
#1517=CYLINDRICAL_SURFACE('',#6848,3.0735);
#1518=CYLINDRICAL_SURFACE('',#6849,3.0735);
#1519=CYLINDRICAL_SURFACE('',#6850,3.0735);
#1520=CYLINDRICAL_SURFACE('',#6852,26.9999999999999);
#1521=CYLINDRICAL_SURFACE('',#6855,2.);
#1522=CYLINDRICAL_SURFACE('',#6858,23.0000000000001);
#1523=CYLINDRICAL_SURFACE('',#6861,2.);
#1524=CYLINDRICAL_SURFACE('',#6864,3.0735);
#1525=CYLINDRICAL_SURFACE('',#6867,2.5175);
#1526=CYLINDRICAL_SURFACE('',#6868,3.);
#1527=CYLINDRICAL_SURFACE('',#6871,3.);
#1528=CYLINDRICAL_SURFACE('',#6874,5.);
#1529=CYLINDRICAL_SURFACE('',#6877,6.);
#1530=CYLINDRICAL_SURFACE('',#6879,10.);
#1531=CYLINDRICAL_SURFACE('',#6893,8.);
#1532=CYLINDRICAL_SURFACE('',#6896,6.);
#1533=CYLINDRICAL_SURFACE('',#6898,6.);
#1646=FACE_BOUND('',#2246,.T.);
#1647=FACE_BOUND('',#2254,.T.);
#1648=FACE_BOUND('',#2255,.T.);
#1649=FACE_BOUND('',#2256,.T.);
#1650=FACE_BOUND('',#2257,.T.);
#1651=FACE_BOUND('',#2258,.T.);
#1652=FACE_BOUND('',#2263,.T.);
#1653=FACE_BOUND('',#2264,.T.);
#1654=FACE_BOUND('',#2265,.T.);
#1655=FACE_BOUND('',#2266,.T.);
#1656=FACE_BOUND('',#2267,.T.);
#1830=FACE_OUTER_BOUND('',#2218,.T.);
#1831=FACE_OUTER_BOUND('',#2219,.T.);
#1832=FACE_OUTER_BOUND('',#2220,.T.);
#1833=FACE_OUTER_BOUND('',#2221,.T.);
#1834=FACE_OUTER_BOUND('',#2222,.T.);
#1835=FACE_OUTER_BOUND('',#2223,.T.);
#1836=FACE_OUTER_BOUND('',#2224,.T.);
#1837=FACE_OUTER_BOUND('',#2225,.T.);
#1838=FACE_OUTER_BOUND('',#2226,.T.);
#1839=FACE_OUTER_BOUND('',#2227,.T.);
#1840=FACE_OUTER_BOUND('',#2228,.T.);
#1841=FACE_OUTER_BOUND('',#2229,.T.);
#1842=FACE_OUTER_BOUND('',#2230,.T.);
#1843=FACE_OUTER_BOUND('',#2231,.T.);
#1844=FACE_OUTER_BOUND('',#2232,.T.);
#1845=FACE_OUTER_BOUND('',#2233,.T.);
#1846=FACE_OUTER_BOUND('',#2234,.T.);
#1847=FACE_OUTER_BOUND('',#2235,.T.);
#1848=FACE_OUTER_BOUND('',#2236,.T.);
#1849=FACE_OUTER_BOUND('',#2237,.T.);
#1850=FACE_OUTER_BOUND('',#2238,.T.);
#1851=FACE_OUTER_BOUND('',#2239,.T.);
#1852=FACE_OUTER_BOUND('',#2240,.T.);
#1853=FACE_OUTER_BOUND('',#2241,.T.);
#1854=FACE_OUTER_BOUND('',#2242,.T.);
#1855=FACE_OUTER_BOUND('',#2243,.T.);
#1856=FACE_OUTER_BOUND('',#2244,.T.);
#1857=FACE_OUTER_BOUND('',#2245,.T.);
#1858=FACE_OUTER_BOUND('',#2247,.T.);
#1859=FACE_OUTER_BOUND('',#2248,.T.);
#1860=FACE_OUTER_BOUND('',#2249,.T.);
#1861=FACE_OUTER_BOUND('',#2250,.T.);
#1862=FACE_OUTER_BOUND('',#2251,.T.);
#1863=FACE_OUTER_BOUND('',#2252,.T.);
#1864=FACE_OUTER_BOUND('',#2253,.T.);
#1865=FACE_OUTER_BOUND('',#2259,.T.);
#1866=FACE_OUTER_BOUND('',#2260,.T.);
#1867=FACE_OUTER_BOUND('',#2261,.T.);
#1868=FACE_OUTER_BOUND('',#2262,.T.);
#1869=FACE_OUTER_BOUND('',#2268,.T.);
#1870=FACE_OUTER_BOUND('',#2269,.T.);
#1871=FACE_OUTER_BOUND('',#2270,.T.);
#1872=FACE_OUTER_BOUND('',#2271,.T.);
#1873=FACE_OUTER_BOUND('',#2272,.T.);
#1874=FACE_OUTER_BOUND('',#2273,.T.);
#2218=EDGE_LOOP('',(#4925,#4926,#4927,#4928));
#2219=EDGE_LOOP('',(#4929,#4930,#4931,#4932));
#2220=EDGE_LOOP('',(#4933,#4934,#4935,#4936));
#2221=EDGE_LOOP('',(#4937,#4938,#4939,#4940));
#2222=EDGE_LOOP('',(#4941,#4942,#4943,#4944));
#2223=EDGE_LOOP('',(#4945,#4946,#4947,#4948));
#2224=EDGE_LOOP('',(#4949,#4950,#4951,#4952));
#2225=EDGE_LOOP('',(#4953,#4954,#4955,#4956));
#2226=EDGE_LOOP('',(#4957,#4958,#4959,#4960));
#2227=EDGE_LOOP('',(#4961,#4962,#4963,#4964));
#2228=EDGE_LOOP('',(#4965,#4966,#4967,#4968));
#2229=EDGE_LOOP('',(#4969,#4970,#4971,#4972));
#2230=EDGE_LOOP('',(#4973,#4974,#4975,#4976));
#2231=EDGE_LOOP('',(#4977,#4978,#4979,#4980));
#2232=EDGE_LOOP('',(#4981,#4982,#4983,#4984));
#2233=EDGE_LOOP('',(#4985,#4986,#4987,#4988));
#2234=EDGE_LOOP('',(#4989,#4990,#4991,#4992));
#2235=EDGE_LOOP('',(#4993,#4994,#4995,#4996));
#2236=EDGE_LOOP('',(#4997,#4998,#4999,#5000));
#2237=EDGE_LOOP('',(#5001,#5002,#5003,#5004));
#2238=EDGE_LOOP('',(#5005,#5006,#5007,#5008));
#2239=EDGE_LOOP('',(#5009,#5010,#5011,#5012));
#2240=EDGE_LOOP('',(#5013,#5014,#5015,#5016));
#2241=EDGE_LOOP('',(#5017,#5018,#5019,#5020));
#2242=EDGE_LOOP('',(#5021,#5022,#5023,#5024));
#2243=EDGE_LOOP('',(#5025,#5026,#5027,#5028,#5029,#5030,#5031,#5032,#5033,
#5034,#5035,#5036,#5037,#5038,#5039,#5040,#5041,#5042,#5043,#5044,#5045,
#5046,#5047,#5048));
#2244=EDGE_LOOP('',(#5049,#5050,#5051,#5052,#5053,#5054,#5055,#5056,#5057,
#5058,#5059,#5060,#5061,#5062,#5063,#5064,#5065,#5066,#5067,#5068,#5069,
#5070,#5071,#5072));
#2245=EDGE_LOOP('',(#5073));
#2246=EDGE_LOOP('',(#5074,#5075,#5076,#5077));
#2247=EDGE_LOOP('',(#5078,#5079,#5080,#5081));
#2248=EDGE_LOOP('',(#5082,#5083,#5084,#5085));
#2249=EDGE_LOOP('',(#5086,#5087,#5088,#5089));
#2250=EDGE_LOOP('',(#5090,#5091,#5092,#5093));
#2251=EDGE_LOOP('',(#5094,#5095,#5096,#5097));
#2252=EDGE_LOOP('',(#5098,#5099,#5100,#5101));
#2253=EDGE_LOOP('',(#5102,#5103,#5104,#5105,#5106,#5107,#5108,#5109,#5110,
#5111));
#2254=EDGE_LOOP('',(#5112,#5113,#5114,#5115));
#2255=EDGE_LOOP('',(#5116));
#2256=EDGE_LOOP('',(#5117));
#2257=EDGE_LOOP('',(#5118));
#2258=EDGE_LOOP('',(#5119));
#2259=EDGE_LOOP('',(#5120,#5121,#5122,#5123));
#2260=EDGE_LOOP('',(#5124,#5125,#5126,#5127));
#2261=EDGE_LOOP('',(#5128,#5129,#5130,#5131));
#2262=EDGE_LOOP('',(#5132,#5133,#5134,#5135,#5136,#5137,#5138,#5139,#5140,
#5141));
#2263=EDGE_LOOP('',(#5142,#5143,#5144,#5145));
#2264=EDGE_LOOP('',(#5146,#5147,#5148,#5149));
#2265=EDGE_LOOP('',(#5150));
#2266=EDGE_LOOP('',(#5151));
#2267=EDGE_LOOP('',(#5152));
#2268=EDGE_LOOP('',(#5153,#5154,#5155,#5156));
#2269=EDGE_LOOP('',(#5157,#5158,#5159,#5160));
#2270=EDGE_LOOP('',(#5161,#5162,#5163,#5164));
#2271=EDGE_LOOP('',(#5165,#5166,#5167,#5168));
#2272=EDGE_LOOP('',(#5169,#5170,#5171,#5172));
#2273=EDGE_LOOP('',(#5173,#5174,#5175,#5176));
#2506=CIRCLE('',#6829,2.5175);
#2507=CIRCLE('',#6839,2.5175);
#2508=CIRCLE('',#6841,3.0735);
#2509=CIRCLE('',#6851,3.0735);
#2510=CIRCLE('',#6853,26.9999999999999);
#2511=CIRCLE('',#6854,26.9999999999999);
#2512=CIRCLE('',#6856,2.);
#2513=CIRCLE('',#6857,2.);
#2514=CIRCLE('',#6859,23.0000000000001);
#2515=CIRCLE('',#6860,23.0000000000001);
#2516=CIRCLE('',#6862,2.);
#2517=CIRCLE('',#6863,2.);
#2518=CIRCLE('',#6866,6.);
#2519=CIRCLE('',#6869,3.);
#2520=CIRCLE('',#6870,3.);
#2521=CIRCLE('',#6872,3.);
#2522=CIRCLE('',#6873,3.);
#2523=CIRCLE('',#6875,5.);
#2524=CIRCLE('',#6876,5.);
#2525=CIRCLE('',#6878,6.);
#2526=CIRCLE('',#6880,10.);
#2527=CIRCLE('',#6881,10.);
#2528=CIRCLE('',#6883,6.);
#2529=CIRCLE('',#6884,8.);
#2530=CIRCLE('',#6885,6.);
#2531=CIRCLE('',#6890,6.);
#2532=CIRCLE('',#6891,8.);
#2533=CIRCLE('',#6892,6.);
#2888=VERTEX_POINT('',#13851);
#2889=VERTEX_POINT('',#13852);
#2890=VERTEX_POINT('',#13854);
#2891=VERTEX_POINT('',#13859);
#2892=VERTEX_POINT('',#13872);
#2893=VERTEX_POINT('',#13873);
#2894=VERTEX_POINT('',#13923);
#2895=VERTEX_POINT('',#13924);
#2896=VERTEX_POINT('',#13974);
#2897=VERTEX_POINT('',#13975);
#2898=VERTEX_POINT('',#14022);
#2899=VERTEX_POINT('',#14023);
#2900=VERTEX_POINT('',#14070);
#2901=VERTEX_POINT('',#14071);
#2902=VERTEX_POINT('',#14121);
#2903=VERTEX_POINT('',#14122);
#2904=VERTEX_POINT('',#14172);
#2905=VERTEX_POINT('',#14173);
#2906=VERTEX_POINT('',#14220);
#2907=VERTEX_POINT('',#14221);
#2908=VERTEX_POINT('',#14271);
#2909=VERTEX_POINT('',#14272);
#2910=VERTEX_POINT('',#14274);
#2911=VERTEX_POINT('',#14288);
#2912=VERTEX_POINT('',#14310);
#2913=VERTEX_POINT('',#14311);
#2914=VERTEX_POINT('',#14313);
#2915=VERTEX_POINT('',#14322);
#2916=VERTEX_POINT('',#14334);
#2917=VERTEX_POINT('',#14335);
#2918=VERTEX_POINT('',#14358);
#2919=VERTEX_POINT('',#14359);
#2920=VERTEX_POINT('',#14383);
#2921=VERTEX_POINT('',#14384);
#2922=VERTEX_POINT('',#14407);
#2923=VERTEX_POINT('',#14408);
#2924=VERTEX_POINT('',#14432);
#2925=VERTEX_POINT('',#14433);
#2926=VERTEX_POINT('',#14456);
#2927=VERTEX_POINT('',#14457);
#2928=VERTEX_POINT('',#14481);
#2929=VERTEX_POINT('',#14482);
#2930=VERTEX_POINT('',#14506);
#2931=VERTEX_POINT('',#14507);
#2932=VERTEX_POINT('',#14530);
#2933=VERTEX_POINT('',#14531);
#2934=VERTEX_POINT('',#14533);
#2935=VERTEX_POINT('',#14539);
#2936=VERTEX_POINT('',#14547);
#2937=VERTEX_POINT('',#14548);
#2938=VERTEX_POINT('',#14550);
#2939=VERTEX_POINT('',#14552);
#2940=VERTEX_POINT('',#14556);
#2941=VERTEX_POINT('',#14558);
#2942=VERTEX_POINT('',#14562);
#2943=VERTEX_POINT('',#14564);
#2944=VERTEX_POINT('',#15566);
#2945=VERTEX_POINT('',#15570);
#2946=VERTEX_POINT('',#15572);
#2947=VERTEX_POINT('',#15576);
#2948=VERTEX_POINT('',#15578);
#2949=VERTEX_POINT('',#15582);
#2950=VERTEX_POINT('',#15584);
#2951=VERTEX_POINT('',#15588);
#2952=VERTEX_POINT('',#15592);
#2953=VERTEX_POINT('',#15593);
#2954=VERTEX_POINT('',#15595);
#2955=VERTEX_POINT('',#15597);
#2956=VERTEX_POINT('',#15601);
#2957=VERTEX_POINT('',#15603);
#2958=VERTEX_POINT('',#15605);
#2959=VERTEX_POINT('',#15607);
#2960=VERTEX_POINT('',#15609);
#2961=VERTEX_POINT('',#15611);
#2962=VERTEX_POINT('',#15613);
#2963=VERTEX_POINT('',#15615);
#2964=VERTEX_POINT('',#15619);
#2965=VERTEX_POINT('',#15623);
#2966=VERTEX_POINT('',#15627);
#2967=VERTEX_POINT('',#15631);
#2968=VERTEX_POINT('',#15633);
#2969=VERTEX_POINT('',#15635);
#2970=VERTEX_POINT('',#15637);
#2971=VERTEX_POINT('',#15639);
#3621=EDGE_CURVE('',#2888,#2889,#724,.T.);
#3622=EDGE_CURVE('',#2889,#2890,#269,.T.);
#3623=EDGE_CURVE('',#2891,#2890,#2506,.F.);
#3624=EDGE_CURVE('',#2891,#2888,#270,.T.);
#3625=EDGE_CURVE('',#2892,#2893,#725,.T.);
#3626=EDGE_CURVE('',#2893,#2889,#271,.T.);
#3627=EDGE_CURVE('',#2888,#2892,#272,.T.);
#3628=EDGE_CURVE('',#2894,#2895,#726,.T.);
#3629=EDGE_CURVE('',#2895,#2893,#273,.T.);
#3630=EDGE_CURVE('',#2892,#2894,#274,.T.);
#3631=EDGE_CURVE('',#2896,#2897,#727,.T.);
#3632=EDGE_CURVE('',#2897,#2895,#275,.T.);
#3633=EDGE_CURVE('',#2894,#2896,#276,.T.);
#3634=EDGE_CURVE('',#2898,#2899,#728,.T.);
#3635=EDGE_CURVE('',#2899,#2897,#277,.T.);
#3636=EDGE_CURVE('',#2896,#2898,#278,.T.);
#3637=EDGE_CURVE('',#2900,#2901,#729,.T.);
#3638=EDGE_CURVE('',#2901,#2899,#279,.T.);
#3639=EDGE_CURVE('',#2898,#2900,#280,.T.);
#3640=EDGE_CURVE('',#2902,#2903,#730,.T.);
#3641=EDGE_CURVE('',#2903,#2901,#281,.T.);
#3642=EDGE_CURVE('',#2900,#2902,#282,.T.);
#3643=EDGE_CURVE('',#2904,#2905,#731,.T.);
#3644=EDGE_CURVE('',#2905,#2903,#283,.T.);
#3645=EDGE_CURVE('',#2902,#2904,#284,.T.);
#3646=EDGE_CURVE('',#2906,#2907,#732,.T.);
#3647=EDGE_CURVE('',#2907,#2905,#285,.T.);
#3648=EDGE_CURVE('',#2904,#2906,#286,.T.);
#3649=EDGE_CURVE('',#2908,#2909,#733,.T.);
#3650=EDGE_CURVE('',#2908,#2910,#287,.T.);
#3651=EDGE_CURVE('',#2911,#2910,#2507,.T.);
#3652=EDGE_CURVE('',#2911,#2909,#288,.T.);
#3653=EDGE_CURVE('',#2912,#2913,#734,.T.);
#3654=EDGE_CURVE('',#2913,#2914,#289,.T.);
#3655=EDGE_CURVE('',#2915,#2914,#2508,.T.);
#3656=EDGE_CURVE('',#2912,#2915,#290,.T.);
#3657=EDGE_CURVE('',#2916,#2917,#735,.T.);
#3658=EDGE_CURVE('',#2917,#2913,#291,.T.);
#3659=EDGE_CURVE('',#2916,#2912,#292,.T.);
#3660=EDGE_CURVE('',#2918,#2919,#736,.T.);
#3661=EDGE_CURVE('',#2919,#2917,#293,.T.);
#3662=EDGE_CURVE('',#2918,#2916,#294,.T.);
#3663=EDGE_CURVE('',#2920,#2921,#737,.T.);
#3664=EDGE_CURVE('',#2921,#2919,#295,.T.);
#3665=EDGE_CURVE('',#2920,#2918,#296,.T.);
#3666=EDGE_CURVE('',#2922,#2923,#738,.T.);
#3667=EDGE_CURVE('',#2923,#2921,#297,.T.);
#3668=EDGE_CURVE('',#2922,#2920,#298,.T.);
#3669=EDGE_CURVE('',#2924,#2925,#739,.T.);
#3670=EDGE_CURVE('',#2925,#2923,#299,.T.);
#3671=EDGE_CURVE('',#2924,#2922,#300,.T.);
#3672=EDGE_CURVE('',#2926,#2927,#740,.T.);
#3673=EDGE_CURVE('',#2927,#2925,#301,.T.);
#3674=EDGE_CURVE('',#2926,#2924,#302,.T.);
#3675=EDGE_CURVE('',#2928,#2929,#741,.T.);
#3676=EDGE_CURVE('',#2929,#2927,#303,.T.);
#3677=EDGE_CURVE('',#2928,#2926,#304,.T.);
#3678=EDGE_CURVE('',#2930,#2931,#742,.T.);
#3679=EDGE_CURVE('',#2931,#2929,#305,.T.);
#3680=EDGE_CURVE('',#2930,#2928,#306,.T.);
#3681=EDGE_CURVE('',#2932,#2933,#743,.T.);
#3682=EDGE_CURVE('',#2934,#2932,#307,.T.);
#3683=EDGE_CURVE('',#2935,#2934,#2509,.T.);
#3684=EDGE_CURVE('',#2935,#2933,#308,.T.);
#3685=EDGE_CURVE('',#2936,#2937,#2510,.T.);
#3686=EDGE_CURVE('',#2936,#2938,#744,.T.);
#3687=EDGE_CURVE('',#2939,#2938,#2511,.T.);
#3688=EDGE_CURVE('',#2937,#2939,#745,.T.);
#3689=EDGE_CURVE('',#2940,#2936,#2512,.T.);
#3690=EDGE_CURVE('',#2940,#2941,#746,.T.);
#3691=EDGE_CURVE('',#2938,#2941,#2513,.T.);
#3692=EDGE_CURVE('',#2942,#2940,#2514,.T.);
#3693=EDGE_CURVE('',#2942,#2943,#747,.T.);
#3694=EDGE_CURVE('',#2941,#2943,#2515,.T.);
#3695=EDGE_CURVE('',#2937,#2942,#2516,.T.);
#3696=EDGE_CURVE('',#2943,#2939,#2517,.T.);
#3697=EDGE_CURVE('',#2933,#2931,#309,.T.);
#3698=EDGE_CURVE('',#2932,#2930,#310,.T.);
#3699=EDGE_CURVE('',#2914,#2891,#311,.T.);
#3700=EDGE_CURVE('',#2910,#2935,#312,.T.);
#3701=EDGE_CURVE('',#2906,#2908,#313,.T.);
#3702=EDGE_CURVE('',#2890,#2915,#314,.T.);
#3703=EDGE_CURVE('',#2909,#2907,#315,.T.);
#3704=EDGE_CURVE('',#2934,#2911,#316,.T.);
#3705=EDGE_CURVE('',#2944,#2944,#2518,.T.);
#3706=EDGE_CURVE('',#2945,#2945,#2519,.T.);
#3707=EDGE_CURVE('',#2945,#2946,#748,.T.);
#3708=EDGE_CURVE('',#2946,#2946,#2520,.T.);
#3709=EDGE_CURVE('',#2947,#2947,#2521,.T.);
#3710=EDGE_CURVE('',#2947,#2948,#749,.T.);
#3711=EDGE_CURVE('',#2948,#2948,#2522,.T.);
#3712=EDGE_CURVE('',#2949,#2949,#2523,.T.);
#3713=EDGE_CURVE('',#2949,#2950,#750,.T.);
#3714=EDGE_CURVE('',#2950,#2950,#2524,.T.);
#3715=EDGE_CURVE('',#2944,#2951,#751,.T.);
#3716=EDGE_CURVE('',#2951,#2951,#2525,.T.);
#3717=EDGE_CURVE('',#2952,#2953,#752,.T.);
#3718=EDGE_CURVE('',#2952,#2954,#2526,.T.);
#3719=EDGE_CURVE('',#2954,#2955,#753,.T.);
#3720=EDGE_CURVE('',#2953,#2955,#2527,.T.);
#3721=EDGE_CURVE('',#2955,#2956,#754,.T.);
#3722=EDGE_CURVE('',#2956,#2957,#755,.T.);
#3723=EDGE_CURVE('',#2957,#2958,#2528,.T.);
#3724=EDGE_CURVE('',#2958,#2959,#756,.T.);
#3725=EDGE_CURVE('',#2959,#2960,#2529,.T.);
#3726=EDGE_CURVE('',#2960,#2961,#757,.T.);
#3727=EDGE_CURVE('',#2961,#2962,#2530,.T.);
#3728=EDGE_CURVE('',#2962,#2963,#758,.T.);
#3729=EDGE_CURVE('',#2963,#2953,#759,.T.);
#3730=EDGE_CURVE('',#2964,#2963,#760,.T.);
#3731=EDGE_CURVE('',#2964,#2952,#761,.T.);
#3732=EDGE_CURVE('',#2956,#2965,#762,.T.);
#3733=EDGE_CURVE('',#2954,#2965,#763,.T.);
#3734=EDGE_CURVE('',#2965,#2966,#764,.T.);
#3735=EDGE_CURVE('',#2966,#2957,#765,.T.);
#3736=EDGE_CURVE('',#2967,#2964,#766,.T.);
#3737=EDGE_CURVE('',#2968,#2967,#2531,.T.);
#3738=EDGE_CURVE('',#2969,#2968,#767,.T.);
#3739=EDGE_CURVE('',#2970,#2969,#2532,.T.);
#3740=EDGE_CURVE('',#2971,#2970,#768,.T.);
#3741=EDGE_CURVE('',#2966,#2971,#2533,.T.);
#3742=EDGE_CURVE('',#2960,#2969,#769,.T.);
#3743=EDGE_CURVE('',#2970,#2959,#770,.T.);
#3744=EDGE_CURVE('',#2967,#2962,#771,.T.);
#3745=EDGE_CURVE('',#2971,#2958,#772,.T.);
#3746=EDGE_CURVE('',#2968,#2961,#773,.T.);
#4925=ORIENTED_EDGE('',*,*,#3621,.T.);
#4926=ORIENTED_EDGE('',*,*,#3622,.T.);
#4927=ORIENTED_EDGE('',*,*,#3623,.F.);
#4928=ORIENTED_EDGE('',*,*,#3624,.T.);
#4929=ORIENTED_EDGE('',*,*,#3625,.T.);
#4930=ORIENTED_EDGE('',*,*,#3626,.T.);
#4931=ORIENTED_EDGE('',*,*,#3621,.F.);
#4932=ORIENTED_EDGE('',*,*,#3627,.T.);
#4933=ORIENTED_EDGE('',*,*,#3628,.T.);
#4934=ORIENTED_EDGE('',*,*,#3629,.T.);
#4935=ORIENTED_EDGE('',*,*,#3625,.F.);
#4936=ORIENTED_EDGE('',*,*,#3630,.T.);
#4937=ORIENTED_EDGE('',*,*,#3631,.T.);
#4938=ORIENTED_EDGE('',*,*,#3632,.T.);
#4939=ORIENTED_EDGE('',*,*,#3628,.F.);
#4940=ORIENTED_EDGE('',*,*,#3633,.T.);
#4941=ORIENTED_EDGE('',*,*,#3634,.T.);
#4942=ORIENTED_EDGE('',*,*,#3635,.T.);
#4943=ORIENTED_EDGE('',*,*,#3631,.F.);
#4944=ORIENTED_EDGE('',*,*,#3636,.T.);
#4945=ORIENTED_EDGE('',*,*,#3637,.T.);
#4946=ORIENTED_EDGE('',*,*,#3638,.T.);
#4947=ORIENTED_EDGE('',*,*,#3634,.F.);
#4948=ORIENTED_EDGE('',*,*,#3639,.T.);
#4949=ORIENTED_EDGE('',*,*,#3640,.T.);
#4950=ORIENTED_EDGE('',*,*,#3641,.T.);
#4951=ORIENTED_EDGE('',*,*,#3637,.F.);
#4952=ORIENTED_EDGE('',*,*,#3642,.T.);
#4953=ORIENTED_EDGE('',*,*,#3643,.T.);
#4954=ORIENTED_EDGE('',*,*,#3644,.T.);
#4955=ORIENTED_EDGE('',*,*,#3640,.F.);
#4956=ORIENTED_EDGE('',*,*,#3645,.T.);
#4957=ORIENTED_EDGE('',*,*,#3646,.T.);
#4958=ORIENTED_EDGE('',*,*,#3647,.T.);
#4959=ORIENTED_EDGE('',*,*,#3643,.F.);
#4960=ORIENTED_EDGE('',*,*,#3648,.T.);
#4961=ORIENTED_EDGE('',*,*,#3649,.F.);
#4962=ORIENTED_EDGE('',*,*,#3650,.T.);
#4963=ORIENTED_EDGE('',*,*,#3651,.F.);
#4964=ORIENTED_EDGE('',*,*,#3652,.T.);
#4965=ORIENTED_EDGE('',*,*,#3653,.T.);
#4966=ORIENTED_EDGE('',*,*,#3654,.T.);
#4967=ORIENTED_EDGE('',*,*,#3655,.F.);
#4968=ORIENTED_EDGE('',*,*,#3656,.F.);
#4969=ORIENTED_EDGE('',*,*,#3657,.T.);
#4970=ORIENTED_EDGE('',*,*,#3658,.T.);
#4971=ORIENTED_EDGE('',*,*,#3653,.F.);
#4972=ORIENTED_EDGE('',*,*,#3659,.F.);
#4973=ORIENTED_EDGE('',*,*,#3660,.T.);
#4974=ORIENTED_EDGE('',*,*,#3661,.T.);
#4975=ORIENTED_EDGE('',*,*,#3657,.F.);
#4976=ORIENTED_EDGE('',*,*,#3662,.F.);
#4977=ORIENTED_EDGE('',*,*,#3663,.T.);
#4978=ORIENTED_EDGE('',*,*,#3664,.T.);
#4979=ORIENTED_EDGE('',*,*,#3660,.F.);
#4980=ORIENTED_EDGE('',*,*,#3665,.F.);
#4981=ORIENTED_EDGE('',*,*,#3666,.T.);
#4982=ORIENTED_EDGE('',*,*,#3667,.T.);
#4983=ORIENTED_EDGE('',*,*,#3663,.F.);
#4984=ORIENTED_EDGE('',*,*,#3668,.F.);
#4985=ORIENTED_EDGE('',*,*,#3669,.T.);
#4986=ORIENTED_EDGE('',*,*,#3670,.T.);
#4987=ORIENTED_EDGE('',*,*,#3666,.F.);
#4988=ORIENTED_EDGE('',*,*,#3671,.F.);
#4989=ORIENTED_EDGE('',*,*,#3672,.T.);
#4990=ORIENTED_EDGE('',*,*,#3673,.T.);
#4991=ORIENTED_EDGE('',*,*,#3669,.F.);
#4992=ORIENTED_EDGE('',*,*,#3674,.F.);
#4993=ORIENTED_EDGE('',*,*,#3675,.T.);
#4994=ORIENTED_EDGE('',*,*,#3676,.T.);
#4995=ORIENTED_EDGE('',*,*,#3672,.F.);
#4996=ORIENTED_EDGE('',*,*,#3677,.F.);
#4997=ORIENTED_EDGE('',*,*,#3678,.T.);
#4998=ORIENTED_EDGE('',*,*,#3679,.T.);
#4999=ORIENTED_EDGE('',*,*,#3675,.F.);
#5000=ORIENTED_EDGE('',*,*,#3680,.F.);
#5001=ORIENTED_EDGE('',*,*,#3681,.F.);
#5002=ORIENTED_EDGE('',*,*,#3682,.F.);
#5003=ORIENTED_EDGE('',*,*,#3683,.F.);
#5004=ORIENTED_EDGE('',*,*,#3684,.T.);
#5005=ORIENTED_EDGE('',*,*,#3685,.F.);
#5006=ORIENTED_EDGE('',*,*,#3686,.T.);
#5007=ORIENTED_EDGE('',*,*,#3687,.F.);
#5008=ORIENTED_EDGE('',*,*,#3688,.F.);
#5009=ORIENTED_EDGE('',*,*,#3689,.F.);
#5010=ORIENTED_EDGE('',*,*,#3690,.T.);
#5011=ORIENTED_EDGE('',*,*,#3691,.F.);
#5012=ORIENTED_EDGE('',*,*,#3686,.F.);
#5013=ORIENTED_EDGE('',*,*,#3692,.F.);
#5014=ORIENTED_EDGE('',*,*,#3693,.T.);
#5015=ORIENTED_EDGE('',*,*,#3694,.F.);
#5016=ORIENTED_EDGE('',*,*,#3690,.F.);
#5017=ORIENTED_EDGE('',*,*,#3695,.F.);
#5018=ORIENTED_EDGE('',*,*,#3688,.T.);
#5019=ORIENTED_EDGE('',*,*,#3696,.F.);
#5020=ORIENTED_EDGE('',*,*,#3693,.F.);
#5021=ORIENTED_EDGE('',*,*,#3681,.T.);
#5022=ORIENTED_EDGE('',*,*,#3697,.T.);
#5023=ORIENTED_EDGE('',*,*,#3678,.F.);
#5024=ORIENTED_EDGE('',*,*,#3698,.F.);
#5025=ORIENTED_EDGE('',*,*,#3699,.F.);
#5026=ORIENTED_EDGE('',*,*,#3654,.F.);
#5027=ORIENTED_EDGE('',*,*,#3658,.F.);
#5028=ORIENTED_EDGE('',*,*,#3661,.F.);
#5029=ORIENTED_EDGE('',*,*,#3664,.F.);
#5030=ORIENTED_EDGE('',*,*,#3667,.F.);
#5031=ORIENTED_EDGE('',*,*,#3670,.F.);
#5032=ORIENTED_EDGE('',*,*,#3673,.F.);
#5033=ORIENTED_EDGE('',*,*,#3676,.F.);
#5034=ORIENTED_EDGE('',*,*,#3679,.F.);
#5035=ORIENTED_EDGE('',*,*,#3697,.F.);
#5036=ORIENTED_EDGE('',*,*,#3684,.F.);
#5037=ORIENTED_EDGE('',*,*,#3700,.F.);
#5038=ORIENTED_EDGE('',*,*,#3650,.F.);
#5039=ORIENTED_EDGE('',*,*,#3701,.F.);
#5040=ORIENTED_EDGE('',*,*,#3648,.F.);
#5041=ORIENTED_EDGE('',*,*,#3645,.F.);
#5042=ORIENTED_EDGE('',*,*,#3642,.F.);
#5043=ORIENTED_EDGE('',*,*,#3639,.F.);
#5044=ORIENTED_EDGE('',*,*,#3636,.F.);
#5045=ORIENTED_EDGE('',*,*,#3633,.F.);
#5046=ORIENTED_EDGE('',*,*,#3630,.F.);
#5047=ORIENTED_EDGE('',*,*,#3627,.F.);
#5048=ORIENTED_EDGE('',*,*,#3624,.F.);
#5049=ORIENTED_EDGE('',*,*,#3702,.F.);
#5050=ORIENTED_EDGE('',*,*,#3622,.F.);
#5051=ORIENTED_EDGE('',*,*,#3626,.F.);
#5052=ORIENTED_EDGE('',*,*,#3629,.F.);
#5053=ORIENTED_EDGE('',*,*,#3632,.F.);
#5054=ORIENTED_EDGE('',*,*,#3635,.F.);
#5055=ORIENTED_EDGE('',*,*,#3638,.F.);
#5056=ORIENTED_EDGE('',*,*,#3641,.F.);
#5057=ORIENTED_EDGE('',*,*,#3644,.F.);
#5058=ORIENTED_EDGE('',*,*,#3647,.F.);
#5059=ORIENTED_EDGE('',*,*,#3703,.F.);
#5060=ORIENTED_EDGE('',*,*,#3652,.F.);
#5061=ORIENTED_EDGE('',*,*,#3704,.F.);
#5062=ORIENTED_EDGE('',*,*,#3682,.T.);
#5063=ORIENTED_EDGE('',*,*,#3698,.T.);
#5064=ORIENTED_EDGE('',*,*,#3680,.T.);
#5065=ORIENTED_EDGE('',*,*,#3677,.T.);
#5066=ORIENTED_EDGE('',*,*,#3674,.T.);
#5067=ORIENTED_EDGE('',*,*,#3671,.T.);
#5068=ORIENTED_EDGE('',*,*,#3668,.T.);
#5069=ORIENTED_EDGE('',*,*,#3665,.T.);
#5070=ORIENTED_EDGE('',*,*,#3662,.T.);
#5071=ORIENTED_EDGE('',*,*,#3659,.T.);
#5072=ORIENTED_EDGE('',*,*,#3656,.T.);
#5073=ORIENTED_EDGE('',*,*,#3705,.T.);
#5074=ORIENTED_EDGE('',*,*,#3700,.T.);
#5075=ORIENTED_EDGE('',*,*,#3683,.T.);
#5076=ORIENTED_EDGE('',*,*,#3704,.T.);
#5077=ORIENTED_EDGE('',*,*,#3651,.T.);
#5078=ORIENTED_EDGE('',*,*,#3649,.T.);
#5079=ORIENTED_EDGE('',*,*,#3703,.T.);
#5080=ORIENTED_EDGE('',*,*,#3646,.F.);
#5081=ORIENTED_EDGE('',*,*,#3701,.T.);
#5082=ORIENTED_EDGE('',*,*,#3706,.F.);
#5083=ORIENTED_EDGE('',*,*,#3707,.T.);
#5084=ORIENTED_EDGE('',*,*,#3708,.F.);
#5085=ORIENTED_EDGE('',*,*,#3707,.F.);
#5086=ORIENTED_EDGE('',*,*,#3709,.F.);
#5087=ORIENTED_EDGE('',*,*,#3710,.T.);
#5088=ORIENTED_EDGE('',*,*,#3711,.F.);
#5089=ORIENTED_EDGE('',*,*,#3710,.F.);
#5090=ORIENTED_EDGE('',*,*,#3712,.F.);
#5091=ORIENTED_EDGE('',*,*,#3713,.T.);
#5092=ORIENTED_EDGE('',*,*,#3714,.F.);
#5093=ORIENTED_EDGE('',*,*,#3713,.F.);
#5094=ORIENTED_EDGE('',*,*,#3705,.F.);
#5095=ORIENTED_EDGE('',*,*,#3715,.T.);
#5096=ORIENTED_EDGE('',*,*,#3716,.F.);
#5097=ORIENTED_EDGE('',*,*,#3715,.F.);
#5098=ORIENTED_EDGE('',*,*,#3717,.F.);
#5099=ORIENTED_EDGE('',*,*,#3718,.T.);
#5100=ORIENTED_EDGE('',*,*,#3719,.T.);
#5101=ORIENTED_EDGE('',*,*,#3720,.F.);
#5102=ORIENTED_EDGE('',*,*,#3721,.T.);
#5103=ORIENTED_EDGE('',*,*,#3722,.T.);
#5104=ORIENTED_EDGE('',*,*,#3723,.T.);
#5105=ORIENTED_EDGE('',*,*,#3724,.T.);
#5106=ORIENTED_EDGE('',*,*,#3725,.T.);
#5107=ORIENTED_EDGE('',*,*,#3726,.T.);
#5108=ORIENTED_EDGE('',*,*,#3727,.T.);
#5109=ORIENTED_EDGE('',*,*,#3728,.T.);
#5110=ORIENTED_EDGE('',*,*,#3729,.T.);
#5111=ORIENTED_EDGE('',*,*,#3720,.T.);
#5112=ORIENTED_EDGE('',*,*,#3685,.T.);
#5113=ORIENTED_EDGE('',*,*,#3695,.T.);
#5114=ORIENTED_EDGE('',*,*,#3692,.T.);
#5115=ORIENTED_EDGE('',*,*,#3689,.T.);
#5116=ORIENTED_EDGE('',*,*,#3706,.T.);
#5117=ORIENTED_EDGE('',*,*,#3709,.T.);
#5118=ORIENTED_EDGE('',*,*,#3712,.T.);
#5119=ORIENTED_EDGE('',*,*,#3716,.T.);
#5120=ORIENTED_EDGE('',*,*,#3730,.F.);
#5121=ORIENTED_EDGE('',*,*,#3731,.T.);
#5122=ORIENTED_EDGE('',*,*,#3717,.T.);
#5123=ORIENTED_EDGE('',*,*,#3729,.F.);
#5124=ORIENTED_EDGE('',*,*,#3732,.F.);
#5125=ORIENTED_EDGE('',*,*,#3721,.F.);
#5126=ORIENTED_EDGE('',*,*,#3719,.F.);
#5127=ORIENTED_EDGE('',*,*,#3733,.T.);
#5128=ORIENTED_EDGE('',*,*,#3732,.T.);
#5129=ORIENTED_EDGE('',*,*,#3734,.T.);
#5130=ORIENTED_EDGE('',*,*,#3735,.T.);
#5131=ORIENTED_EDGE('',*,*,#3722,.F.);
#5132=ORIENTED_EDGE('',*,*,#3731,.F.);
#5133=ORIENTED_EDGE('',*,*,#3736,.F.);
#5134=ORIENTED_EDGE('',*,*,#3737,.F.);
#5135=ORIENTED_EDGE('',*,*,#3738,.F.);
#5136=ORIENTED_EDGE('',*,*,#3739,.F.);
#5137=ORIENTED_EDGE('',*,*,#3740,.F.);
#5138=ORIENTED_EDGE('',*,*,#3741,.F.);
#5139=ORIENTED_EDGE('',*,*,#3734,.F.);
#5140=ORIENTED_EDGE('',*,*,#3733,.F.);
#5141=ORIENTED_EDGE('',*,*,#3718,.F.);
#5142=ORIENTED_EDGE('',*,*,#3687,.T.);
#5143=ORIENTED_EDGE('',*,*,#3691,.T.);
#5144=ORIENTED_EDGE('',*,*,#3694,.T.);
#5145=ORIENTED_EDGE('',*,*,#3696,.T.);
#5146=ORIENTED_EDGE('',*,*,#3699,.T.);
#5147=ORIENTED_EDGE('',*,*,#3623,.T.);
#5148=ORIENTED_EDGE('',*,*,#3702,.T.);
#5149=ORIENTED_EDGE('',*,*,#3655,.T.);
#5150=ORIENTED_EDGE('',*,*,#3708,.T.);
#5151=ORIENTED_EDGE('',*,*,#3711,.T.);
#5152=ORIENTED_EDGE('',*,*,#3714,.T.);
#5153=ORIENTED_EDGE('',*,*,#3742,.F.);
#5154=ORIENTED_EDGE('',*,*,#3725,.F.);
#5155=ORIENTED_EDGE('',*,*,#3743,.F.);
#5156=ORIENTED_EDGE('',*,*,#3739,.T.);
#5157=ORIENTED_EDGE('',*,*,#3730,.T.);
#5158=ORIENTED_EDGE('',*,*,#3728,.F.);
#5159=ORIENTED_EDGE('',*,*,#3744,.F.);
#5160=ORIENTED_EDGE('',*,*,#3736,.T.);
#5161=ORIENTED_EDGE('',*,*,#3743,.T.);
#5162=ORIENTED_EDGE('',*,*,#3724,.F.);
#5163=ORIENTED_EDGE('',*,*,#3745,.F.);
#5164=ORIENTED_EDGE('',*,*,#3740,.T.);
#5165=ORIENTED_EDGE('',*,*,#3737,.T.);
#5166=ORIENTED_EDGE('',*,*,#3744,.T.);
#5167=ORIENTED_EDGE('',*,*,#3727,.F.);
#5168=ORIENTED_EDGE('',*,*,#3746,.F.);
#5169=ORIENTED_EDGE('',*,*,#3742,.T.);
#5170=ORIENTED_EDGE('',*,*,#3738,.T.);
#5171=ORIENTED_EDGE('',*,*,#3746,.T.);
#5172=ORIENTED_EDGE('',*,*,#3726,.F.);
#5173=ORIENTED_EDGE('',*,*,#3741,.T.);
#5174=ORIENTED_EDGE('',*,*,#3745,.T.);
#5175=ORIENTED_EDGE('',*,*,#3723,.F.);
#5176=ORIENTED_EDGE('',*,*,#3735,.F.);
#5975=PLANE('',#6865);
#5976=PLANE('',#6882);
#5977=PLANE('',#6886);
#5978=PLANE('',#6887);
#5979=PLANE('',#6888);
#5980=PLANE('',#6889);
#5981=PLANE('',#6894);
#5982=PLANE('',#6895);
#5983=PLANE('',#6897);
#6209=ADVANCED_FACE('',(#1830),#1500,.F.);
#6210=ADVANCED_FACE('',(#1831),#1501,.F.);
#6211=ADVANCED_FACE('',(#1832),#1502,.F.);
#6212=ADVANCED_FACE('',(#1833),#1503,.F.);
#6213=ADVANCED_FACE('',(#1834),#1504,.F.);
#6214=ADVANCED_FACE('',(#1835),#1505,.F.);
#6215=ADVANCED_FACE('',(#1836),#1506,.F.);
#6216=ADVANCED_FACE('',(#1837),#1507,.F.);
#6217=ADVANCED_FACE('',(#1838),#1508,.F.);
#6218=ADVANCED_FACE('',(#1839),#1509,.F.);
#6219=ADVANCED_FACE('',(#1840),#1510,.F.);
#6220=ADVANCED_FACE('',(#1841),#1511,.F.);
#6221=ADVANCED_FACE('',(#1842),#1512,.F.);
#6222=ADVANCED_FACE('',(#1843),#1513,.F.);
#6223=ADVANCED_FACE('',(#1844),#1514,.F.);
#6224=ADVANCED_FACE('',(#1845),#1515,.F.);
#6225=ADVANCED_FACE('',(#1846),#1516,.F.);
#6226=ADVANCED_FACE('',(#1847),#1517,.F.);
#6227=ADVANCED_FACE('',(#1848),#1518,.F.);
#6228=ADVANCED_FACE('',(#1849),#1519,.F.);
#6229=ADVANCED_FACE('',(#1850),#1520,.F.);
#6230=ADVANCED_FACE('',(#1851),#1521,.F.);
#6231=ADVANCED_FACE('',(#1852),#1522,.T.);
#6232=ADVANCED_FACE('',(#1853),#1523,.F.);
#6233=ADVANCED_FACE('',(#1854),#1524,.F.);
#6234=ADVANCED_FACE('',(#1855),#121,.F.);
#6235=ADVANCED_FACE('',(#1856),#122,.F.);
#6236=ADVANCED_FACE('',(#1857,#1646),#5975,.T.);
#6237=ADVANCED_FACE('',(#1858),#1525,.F.);
#6238=ADVANCED_FACE('',(#1859),#1526,.F.);
#6239=ADVANCED_FACE('',(#1860),#1527,.F.);
#6240=ADVANCED_FACE('',(#1861),#1528,.F.);
#6241=ADVANCED_FACE('',(#1862),#1529,.T.);
#6242=ADVANCED_FACE('',(#1863),#1530,.T.);
#6243=ADVANCED_FACE('',(#1864,#1647,#1648,#1649,#1650,#1651),#5976,.T.);
#6244=ADVANCED_FACE('',(#1865),#5977,.T.);
#6245=ADVANCED_FACE('',(#1866),#5978,.T.);
#6246=ADVANCED_FACE('',(#1867),#5979,.T.);
#6247=ADVANCED_FACE('',(#1868,#1652,#1653,#1654,#1655,#1656),#5980,.F.);
#6248=ADVANCED_FACE('',(#1869),#1531,.T.);
#6249=ADVANCED_FACE('',(#1870),#5981,.T.);
#6250=ADVANCED_FACE('',(#1871),#5982,.T.);
#6251=ADVANCED_FACE('',(#1872),#1532,.T.);
#6252=ADVANCED_FACE('',(#1873),#5983,.T.);
#6253=ADVANCED_FACE('',(#1874),#1533,.T.);
#6426=CLOSED_SHELL('',(#6209,#6210,#6211,#6212,#6213,#6214,#6215,#6216,
#6217,#6218,#6219,#6220,#6221,#6222,#6223,#6224,#6225,#6226,#6227,#6228,
#6229,#6230,#6231,#6232,#6233,#6234,#6235,#6236,#6237,#6238,#6239,#6240,
#6241,#6242,#6243,#6244,#6245,#6246,#6247,#6248,#6249,#6250,#6251,#6252,
#6253));
#6827=AXIS2_PLACEMENT_3D('',#13849,#7770,#7771);
#6828=AXIS2_PLACEMENT_3D('',#13850,#7772,#7773);
#6829=AXIS2_PLACEMENT_3D('',#13860,#7775,#7776);
#6830=AXIS2_PLACEMENT_3D('',#13871,#7777,#7778);
#6831=AXIS2_PLACEMENT_3D('',#13922,#7780,#7781);
#6832=AXIS2_PLACEMENT_3D('',#13973,#7783,#7784);
#6833=AXIS2_PLACEMENT_3D('',#14021,#7786,#7787);
#6834=AXIS2_PLACEMENT_3D('',#14069,#7789,#7790);
#6835=AXIS2_PLACEMENT_3D('',#14120,#7792,#7793);
#6836=AXIS2_PLACEMENT_3D('',#14171,#7795,#7796);
#6837=AXIS2_PLACEMENT_3D('',#14219,#7798,#7799);
#6838=AXIS2_PLACEMENT_3D('',#14270,#7801,#7802);
#6839=AXIS2_PLACEMENT_3D('',#14289,#7804,#7805);
#6840=AXIS2_PLACEMENT_3D('',#14309,#7806,#7807);
#6841=AXIS2_PLACEMENT_3D('',#14323,#7809,#7810);
#6842=AXIS2_PLACEMENT_3D('',#14333,#7811,#7812);
#6843=AXIS2_PLACEMENT_3D('',#14357,#7814,#7815);
#6844=AXIS2_PLACEMENT_3D('',#14382,#7817,#7818);
#6845=AXIS2_PLACEMENT_3D('',#14406,#7820,#7821);
#6846=AXIS2_PLACEMENT_3D('',#14431,#7823,#7824);
#6847=AXIS2_PLACEMENT_3D('',#14455,#7826,#7827);
#6848=AXIS2_PLACEMENT_3D('',#14480,#7829,#7830);
#6849=AXIS2_PLACEMENT_3D('',#14505,#7832,#7833);
#6850=AXIS2_PLACEMENT_3D('',#14529,#7835,#7836);
#6851=AXIS2_PLACEMENT_3D('',#14540,#7838,#7839);
#6852=AXIS2_PLACEMENT_3D('',#14546,#7840,#7841);
#6853=AXIS2_PLACEMENT_3D('',#14549,#7842,#7843);
#6854=AXIS2_PLACEMENT_3D('',#14553,#7845,#7846);
#6855=AXIS2_PLACEMENT_3D('',#14555,#7848,#7849);
#6856=AXIS2_PLACEMENT_3D('',#14557,#7850,#7851);
#6857=AXIS2_PLACEMENT_3D('',#14560,#7853,#7854);
#6858=AXIS2_PLACEMENT_3D('',#14561,#7855,#7856);
#6859=AXIS2_PLACEMENT_3D('',#14563,#7857,#7858);
#6860=AXIS2_PLACEMENT_3D('',#14566,#7860,#7861);
#6861=AXIS2_PLACEMENT_3D('',#14567,#7862,#7863);
#6862=AXIS2_PLACEMENT_3D('',#14568,#7864,#7865);
#6863=AXIS2_PLACEMENT_3D('',#14569,#7866,#7867);
#6864=AXIS2_PLACEMENT_3D('',#14570,#7868,#7869);
#6865=AXIS2_PLACEMENT_3D('',#15565,#7870,#7871);
#6866=AXIS2_PLACEMENT_3D('',#15567,#7872,#7873);
#6867=AXIS2_PLACEMENT_3D('',#15568,#7874,#7875);
#6868=AXIS2_PLACEMENT_3D('',#15569,#7876,#7877);
#6869=AXIS2_PLACEMENT_3D('',#15571,#7878,#7879);
#6870=AXIS2_PLACEMENT_3D('',#15574,#7881,#7882);
#6871=AXIS2_PLACEMENT_3D('',#15575,#7883,#7884);
#6872=AXIS2_PLACEMENT_3D('',#15577,#7885,#7886);
#6873=AXIS2_PLACEMENT_3D('',#15580,#7888,#7889);
#6874=AXIS2_PLACEMENT_3D('',#15581,#7890,#7891);
#6875=AXIS2_PLACEMENT_3D('',#15583,#7892,#7893);
#6876=AXIS2_PLACEMENT_3D('',#15586,#7895,#7896);
#6877=AXIS2_PLACEMENT_3D('',#15587,#7897,#7898);
#6878=AXIS2_PLACEMENT_3D('',#15590,#7900,#7901);
#6879=AXIS2_PLACEMENT_3D('',#15591,#7902,#7903);
#6880=AXIS2_PLACEMENT_3D('',#15596,#7905,#7906);
#6881=AXIS2_PLACEMENT_3D('',#15599,#7908,#7909);
#6882=AXIS2_PLACEMENT_3D('',#15600,#7910,#7911);
#6883=AXIS2_PLACEMENT_3D('',#15606,#7914,#7915);
#6884=AXIS2_PLACEMENT_3D('',#15610,#7917,#7918);
#6885=AXIS2_PLACEMENT_3D('',#15614,#7920,#7921);
#6886=AXIS2_PLACEMENT_3D('',#15618,#7924,#7925);
#6887=AXIS2_PLACEMENT_3D('',#15622,#7928,#7929);
#6888=AXIS2_PLACEMENT_3D('',#15626,#7932,#7933);
#6889=AXIS2_PLACEMENT_3D('',#15630,#7936,#7937);
#6890=AXIS2_PLACEMENT_3D('',#15634,#7939,#7940);
#6891=AXIS2_PLACEMENT_3D('',#15638,#7942,#7943);
#6892=AXIS2_PLACEMENT_3D('',#15641,#7945,#7946);
#6893=AXIS2_PLACEMENT_3D('',#15642,#7947,#7948);
#6894=AXIS2_PLACEMENT_3D('',#15645,#7951,#7952);
#6895=AXIS2_PLACEMENT_3D('',#15647,#7954,#7955);
#6896=AXIS2_PLACEMENT_3D('',#15649,#7957,#7958);
#6897=AXIS2_PLACEMENT_3D('',#15651,#7960,#7961);
#6898=AXIS2_PLACEMENT_3D('',#15652,#7962,#7963);
#7770=DIRECTION('axis',(0.,0.,1.));
#7771=DIRECTION('refdir',(1.,0.,0.));
#7772=DIRECTION('center_axis',(0.,0.,-1.));
#7773=DIRECTION('ref_axis',(-0.346960385471041,0.937879784894517,0.));
#7774=DIRECTION('',(0.,0.,-1.));
#7775=DIRECTION('center_axis',(0.,0.,-1.));
#7776=DIRECTION('ref_axis',(1.,0.,0.));
#7777=DIRECTION('center_axis',(0.,0.,-1.));
#7778=DIRECTION('ref_axis',(1.,0.,0.));
#7779=DIRECTION('',(0.,0.,-1.));
#7780=DIRECTION('center_axis',(0.,0.,-1.));
#7781=DIRECTION('ref_axis',(1.,0.,0.));
#7782=DIRECTION('',(0.,0.,-1.));
#7783=DIRECTION('center_axis',(0.,0.,-1.));
#7784=DIRECTION('ref_axis',(1.,0.,0.));
#7785=DIRECTION('',(0.,0.,-1.));
#7786=DIRECTION('center_axis',(0.,0.,-1.));
#7787=DIRECTION('ref_axis',(1.,0.,0.));
#7788=DIRECTION('',(0.,0.,-1.));
#7789=DIRECTION('center_axis',(0.,0.,-1.));
#7790=DIRECTION('ref_axis',(1.,0.,0.));
#7791=DIRECTION('',(0.,0.,-1.));
#7792=DIRECTION('center_axis',(0.,0.,-1.));
#7793=DIRECTION('ref_axis',(1.,0.,0.));
#7794=DIRECTION('',(0.,0.,-1.));
#7795=DIRECTION('center_axis',(0.,0.,-1.));
#7796=DIRECTION('ref_axis',(1.,0.,0.));
#7797=DIRECTION('',(0.,0.,-1.));
#7798=DIRECTION('center_axis',(0.,0.,-1.));
#7799=DIRECTION('ref_axis',(1.,0.,0.));
#7800=DIRECTION('',(0.,0.,-1.));
#7801=DIRECTION('center_axis',(0.,0.,-1.));
#7802=DIRECTION('ref_axis',(0.937992883095123,-0.346654512826386,0.));
#7803=DIRECTION('',(0.,0.,-1.));
#7804=DIRECTION('center_axis',(0.,0.,-1.));
#7805=DIRECTION('ref_axis',(1.,0.,0.));
#7806=DIRECTION('center_axis',(0.,0.,-1.));
#7807=DIRECTION('ref_axis',(1.,-3.75673318890569E-14,0.));
#7808=DIRECTION('',(1.22464679914735E-16,-4.6156688728706E-30,-1.));
#7809=DIRECTION('center_axis',(0.,0.,1.));
#7810=DIRECTION('ref_axis',(1.,-3.75673318890569E-14,0.));
#7811=DIRECTION('center_axis',(0.,0.,-1.));
#7812=DIRECTION('ref_axis',(1.,-3.75673318890569E-14,0.));
#7813=DIRECTION('',(1.22464679914735E-16,-4.6156688728706E-30,-1.));
#7814=DIRECTION('center_axis',(0.,0.,-1.));
#7815=DIRECTION('ref_axis',(1.,-3.75673318890569E-14,0.));
#7816=DIRECTION('',(1.22464679914735E-16,-4.6156688728706E-30,-1.));
#7817=DIRECTION('center_axis',(0.,0.,-1.));
#7818=DIRECTION('ref_axis',(1.,-3.75673318890569E-14,0.));
#7819=DIRECTION('',(1.22464679914735E-16,-4.6156688728706E-30,-1.));
#7820=DIRECTION('center_axis',(0.,0.,-1.));
#7821=DIRECTION('ref_axis',(1.,-3.75673318890569E-14,0.));
#7822=DIRECTION('',(1.22464679914735E-16,-4.6156688728706E-30,-1.));
#7823=DIRECTION('center_axis',(0.,0.,-1.));
#7824=DIRECTION('ref_axis',(1.,-3.75673318890569E-14,0.));
#7825=DIRECTION('',(1.22464679914735E-16,-4.6156688728706E-30,-1.));
#7826=DIRECTION('center_axis',(0.,0.,-1.));
#7827=DIRECTION('ref_axis',(1.,-3.75673318890569E-14,0.));
#7828=DIRECTION('',(1.22464679914735E-16,-4.6156688728706E-30,-1.));
#7829=DIRECTION('center_axis',(0.,0.,-1.));
#7830=DIRECTION('ref_axis',(1.,-3.75673318890569E-14,0.));
#7831=DIRECTION('',(1.22464679914735E-16,-4.6156688728706E-30,-1.));
#7832=DIRECTION('center_axis',(0.,0.,-1.));
#7833=DIRECTION('ref_axis',(1.,-3.75673318890569E-14,0.));
#7834=DIRECTION('',(1.22464679914735E-16,-4.6156688728706E-30,-1.));
#7835=DIRECTION('center_axis',(0.,0.,-1.));
#7836=DIRECTION('ref_axis',(-0.609232734071224,-0.792991472675527,0.));
#7837=DIRECTION('',(1.22464679914735E-16,-4.6156688728706E-30,-1.));
#7838=DIRECTION('center_axis',(0.,0.,-1.));
#7839=DIRECTION('ref_axis',(1.,-3.75673318890569E-14,0.));
#7840=DIRECTION('center_axis',(0.,0.,-1.));
#7841=DIRECTION('ref_axis',(0.275637355817,0.961261695938319,0.));
#7842=DIRECTION('center_axis',(0.,0.,-1.));
#7843=DIRECTION('ref_axis',(0.275637355817,0.961261695938319,0.));
#7844=DIRECTION('',(0.,0.,-1.));
#7845=DIRECTION('center_axis',(0.,0.,1.));
#7846=DIRECTION('ref_axis',(0.275637355817,0.961261695938319,0.));
#7847=DIRECTION('',(0.,0.,-1.));
#7848=DIRECTION('center_axis',(0.,0.,-1.));
#7849=DIRECTION('ref_axis',(-0.961261693884661,-0.275637362978957,0.));
#7850=DIRECTION('center_axis',(0.,0.,-1.));
#7851=DIRECTION('ref_axis',(-0.275637355816999,0.961261695938319,0.));
#7852=DIRECTION('',(0.,0.,-1.));
#7853=DIRECTION('center_axis',(0.,0.,1.));
#7854=DIRECTION('ref_axis',(-0.275637355816999,0.961261695938319,0.));
#7855=DIRECTION('center_axis',(0.,0.,-1.));
#7856=DIRECTION('ref_axis',(0.275637355816998,0.961261695938319,0.));
#7857=DIRECTION('center_axis',(0.,0.,1.));
#7858=DIRECTION('ref_axis',(0.275637355816998,0.961261695938319,0.));
#7859=DIRECTION('',(0.,0.,-1.));
#7860=DIRECTION('center_axis',(0.,0.,-1.));
#7861=DIRECTION('ref_axis',(0.275637355816998,0.961261695938319,0.));
#7862=DIRECTION('center_axis',(0.,0.,-1.));
#7863=DIRECTION('ref_axis',(-0.275637355817,-0.961261695938319,0.));
#7864=DIRECTION('center_axis',(0.,0.,-1.));
#7865=DIRECTION('ref_axis',(-0.275637355817,-0.961261695938319,0.));
#7866=DIRECTION('center_axis',(0.,0.,1.));
#7867=DIRECTION('ref_axis',(-0.275637355817,-0.961261695938319,0.));
#7868=DIRECTION('center_axis',(0.,0.,-1.));
#7869=DIRECTION('ref_axis',(1.,-3.75673318890569E-14,0.));
#7870=DIRECTION('center_axis',(0.,0.,1.));
#7871=DIRECTION('ref_axis',(1.,0.,0.));
#7872=DIRECTION('center_axis',(0.,0.,1.));
#7873=DIRECTION('ref_axis',(1.,0.,0.));
#7874=DIRECTION('center_axis',(0.,0.,-1.));
#7875=DIRECTION('ref_axis',(1.,0.,0.));
#7876=DIRECTION('center_axis',(0.,0.,-1.));
#7877=DIRECTION('ref_axis',(1.,0.,0.));
#7878=DIRECTION('center_axis',(0.,0.,-1.));
#7879=DIRECTION('ref_axis',(1.,0.,0.));
#7880=DIRECTION('',(0.,0.,-1.));
#7881=DIRECTION('center_axis',(0.,0.,1.));
#7882=DIRECTION('ref_axis',(1.,0.,0.));
#7883=DIRECTION('center_axis',(0.,0.,-1.));
#7884=DIRECTION('ref_axis',(1.,0.,0.));
#7885=DIRECTION('center_axis',(0.,0.,-1.));
#7886=DIRECTION('ref_axis',(1.,0.,0.));
#7887=DIRECTION('',(0.,0.,-1.));
#7888=DIRECTION('center_axis',(0.,0.,1.));
#7889=DIRECTION('ref_axis',(1.,0.,0.));
#7890=DIRECTION('center_axis',(0.,0.,-1.));
#7891=DIRECTION('ref_axis',(1.,0.,0.));
#7892=DIRECTION('center_axis',(0.,0.,-1.));
#7893=DIRECTION('ref_axis',(1.,0.,0.));
#7894=DIRECTION('',(0.,0.,-1.));
#7895=DIRECTION('center_axis',(0.,0.,1.));
#7896=DIRECTION('ref_axis',(1.,0.,0.));
#7897=DIRECTION('center_axis',(0.,0.,1.));
#7898=DIRECTION('ref_axis',(1.,0.,0.));
#7899=DIRECTION('',(0.,0.,-1.));
#7900=DIRECTION('center_axis',(0.,0.,-1.));
#7901=DIRECTION('ref_axis',(1.,0.,0.));
#7902=DIRECTION('center_axis',(0.,0.,1.));
#7903=DIRECTION('ref_axis',(1.,0.,0.));
#7904=DIRECTION('',(0.,0.,1.));
#7905=DIRECTION('center_axis',(0.,0.,1.));
#7906=DIRECTION('ref_axis',(1.,0.,0.));
#7907=DIRECTION('',(0.,0.,1.));
#7908=DIRECTION('center_axis',(0.,0.,1.));
#7909=DIRECTION('ref_axis',(1.,0.,0.));
#7910=DIRECTION('center_axis',(0.,0.,1.));
#7911=DIRECTION('ref_axis',(1.,0.,0.));
#7912=DIRECTION('',(0.,-1.,0.));
#7913=DIRECTION('',(-1.,0.,0.));
#7914=DIRECTION('center_axis',(0.,0.,1.));
#7915=DIRECTION('ref_axis',(0.,1.,0.));
#7916=DIRECTION('',(1.,0.,0.));
#7917=DIRECTION('center_axis',(0.,0.,1.));
#7918=DIRECTION('ref_axis',(1.,0.,0.));
#7919=DIRECTION('',(1.,0.,0.));
#7920=DIRECTION('center_axis',(0.,0.,1.));
#7921=DIRECTION('ref_axis',(0.,-1.,0.));
#7922=DIRECTION('',(-1.,0.,0.));
#7923=DIRECTION('',(0.,1.,0.));
#7924=DIRECTION('center_axis',(1.,0.,0.));
#7925=DIRECTION('ref_axis',(0.,1.,0.));
#7926=DIRECTION('',(0.,0.,1.));
#7927=DIRECTION('',(0.,1.,0.));
#7928=DIRECTION('center_axis',(-1.,0.,0.));
#7929=DIRECTION('ref_axis',(0.,-1.,0.));
#7930=DIRECTION('',(0.,0.,-1.));
#7931=DIRECTION('',(0.,-1.,0.));
#7932=DIRECTION('center_axis',(0.,1.,0.));
#7933=DIRECTION('ref_axis',(-1.,0.,0.));
#7934=DIRECTION('',(-1.,0.,0.));
#7935=DIRECTION('',(0.,0.,1.));
#7936=DIRECTION('center_axis',(0.,0.,1.));
#7937=DIRECTION('ref_axis',(1.,0.,0.));
#7938=DIRECTION('',(-1.,0.,0.));
#7939=DIRECTION('center_axis',(0.,0.,1.));
#7940=DIRECTION('ref_axis',(0.,-1.,0.));
#7941=DIRECTION('',(1.,0.,0.));
#7942=DIRECTION('center_axis',(0.,0.,1.));
#7943=DIRECTION('ref_axis',(1.,0.,0.));
#7944=DIRECTION('',(1.,0.,0.));
#7945=DIRECTION('center_axis',(0.,0.,1.));
#7946=DIRECTION('ref_axis',(0.,1.,0.));
#7947=DIRECTION('center_axis',(0.,0.,1.));
#7948=DIRECTION('ref_axis',(1.,0.,0.));
#7949=DIRECTION('',(0.,0.,-1.));
#7950=DIRECTION('',(0.,0.,1.));
#7951=DIRECTION('center_axis',(0.,1.,0.));
#7952=DIRECTION('ref_axis',(-1.,0.,0.));
#7953=DIRECTION('',(0.,0.,1.));
#7954=DIRECTION('center_axis',(0.,-1.,0.));
#7955=DIRECTION('ref_axis',(1.,0.,0.));
#7956=DIRECTION('',(0.,0.,1.));
#7957=DIRECTION('center_axis',(0.,0.,1.));
#7958=DIRECTION('ref_axis',(0.,-1.,0.));
#7959=DIRECTION('',(0.,0.,1.));
#7960=DIRECTION('center_axis',(0.,-1.,0.));
#7961=DIRECTION('ref_axis',(1.,0.,0.));
#7962=DIRECTION('center_axis',(0.,0.,1.));
#7963=DIRECTION('ref_axis',(0.,1.,0.));
#13849=CARTESIAN_POINT('',(0.,0.,0.));
#13850=CARTESIAN_POINT('Origin',(0.,50.,5.));
#13851=CARTESIAN_POINT('',(-2.51343913234902,50.0006110695374,0.387416697508021));
#13852=CARTESIAN_POINT('',(-2.51566539374153,49.9965492175946,0.112583302491982));
#13853=CARTESIAN_POINT('',(-2.5175,50.,5.));
#13854=CARTESIAN_POINT('',(-1.91346599666504,51.635987203375,0.));
#13855=CARTESIAN_POINT('Ctrl Pts',(-2.51566539374153,49.9965492175946,0.112583302491982));
#13856=CARTESIAN_POINT('Ctrl Pts',(-2.51039880334568,50.5891289186517,0.0750555349946544));
#13857=CARTESIAN_POINT('Ctrl Pts',(-2.29922182808404,51.1848035603044,0.0375277674973273));
#13858=CARTESIAN_POINT('Ctrl Pts',(-1.91346599666504,51.635987203375,0.));
#13859=CARTESIAN_POINT('',(1.91709598686657,51.6387689967411,1.61160490543685E-15));
#13860=CARTESIAN_POINT('Origin',(0.,50.,0.));
#13861=CARTESIAN_POINT('Ctrl Pts',(1.91709858156531,51.6387709851531,1.07542748506512E-15));
#13862=CARTESIAN_POINT('Ctrl Pts',(1.38628707679971,52.2578898930047,0.0517824693358739));
#13863=CARTESIAN_POINT('Ctrl Pts',(0.526694557934675,52.5973407510515,0.103564938671746));
#13864=CARTESIAN_POINT('Ctrl Pts',(-0.283636619336389,52.50549272868,0.155347408007619));
#13865=CARTESIAN_POINT('Ctrl Pts',(-1.11189767700716,52.4116124211116,0.208275647749513));
#13866=CARTESIAN_POINT('Ctrl Pts',(-1.88869330258108,51.8671357122805,0.261203887491408));
#13867=CARTESIAN_POINT('Ctrl Pts',(-2.2589562141896,51.1206233620097,0.314132127233303));
#13868=CARTESIAN_POINT('Ctrl Pts',(-2.42984519203468,50.7760824196498,0.338560317324876));
#13869=CARTESIAN_POINT('Ctrl Pts',(-2.51413710353789,50.3885051034776,0.362988507416448));
#13870=CARTESIAN_POINT('Ctrl Pts',(-2.51343913234902,50.0006110695374,0.387416697508021));
#13871=CARTESIAN_POINT('Origin',(0.,50.,5.));
#13872=CARTESIAN_POINT('',(-2.51733703324273,49.9976965409071,1.38741669750802));
#13873=CARTESIAN_POINT('',(-2.52165773822405,50.0001226503677,1.11258330249199));
#13874=CARTESIAN_POINT('',(-2.5175,50.,5.));
#13875=CARTESIAN_POINT('Ctrl Pts',(-2.52165773822405,50.0001226503677,1.11258330249199));
#13876=CARTESIAN_POINT('Ctrl Pts',(-2.52166128694809,50.005845022657,1.11221987985459));
#13877=CARTESIAN_POINT('Ctrl Pts',(-2.52164349662147,50.0115673701366,1.11185645721719));
#13878=CARTESIAN_POINT('Ctrl Pts',(-2.52160430081332,50.0172895688312,1.11149303457979));
#13879=CARTESIAN_POINT('Ctrl Pts',(-2.51589589160278,50.85066061727,1.05856479483789));
#13880=CARTESIAN_POINT('Ctrl Pts',(-2.05616647103081,51.6808758587515,1.005636555096));
#13881=CARTESIAN_POINT('Ctrl Pts',(-1.35284854651385,52.1280190247019,0.952708315354104));
#13882=CARTESIAN_POINT('Ctrl Pts',(-0.64953062199688,52.5751621906524,0.899780075612209));
#13883=CARTESIAN_POINT('Ctrl Pts',(0.297375806465088,52.6392332810719,0.846851835870316));
#13884=CARTESIAN_POINT('Ctrl Pts',(1.05442258508657,52.2906908988364,0.793923596128421));
#13885=CARTESIAN_POINT('Ctrl Pts',(1.81146936370803,51.9421485166009,0.740995356386527));
#13886=CARTESIAN_POINT('Ctrl Pts',(2.37865649248901,51.1809926617104,0.688067116644633));
#13887=CARTESIAN_POINT('Ctrl Pts',(2.49637754307185,50.3560583642436,0.635138876902739));
#13888=CARTESIAN_POINT('Ctrl Pts',(2.61409859365469,49.5311240667767,0.582210637160844));
#13889=CARTESIAN_POINT('Ctrl Pts',(2.28235356603936,48.6424113267335,0.529282397418948));
#13890=CARTESIAN_POINT('Ctrl Pts',(1.65296007195949,48.0958828038186,0.476354157677053));
#13891=CARTESIAN_POINT('Ctrl Pts',(1.02356657787963,47.5493542809037,0.423425917935159));
#13892=CARTESIAN_POINT('Ctrl Pts',(0.0965246173352477,47.345009975117,0.370497678193264));
#13893=CARTESIAN_POINT('Ctrl Pts',(-0.703763051564332,47.5780837468121,
0.31756943845137));
#13894=CARTESIAN_POINT('Ctrl Pts',(-1.50405072046391,47.8111575185072,0.264641198709475));
#13895=CARTESIAN_POINT('Ctrl Pts',(-2.17758409771868,48.4816493676841,0.21171295896758));
#13896=CARTESIAN_POINT('Ctrl Pts',(-2.41595304962114,49.2787722121955,0.158784719225686));
#13897=CARTESIAN_POINT('Ctrl Pts',(-2.48531100381804,49.51071017768,0.143384246981118));
#13898=CARTESIAN_POINT('Ctrl Pts',(-2.51782667283229,49.7533690913194,0.12798377473655));
#13899=CARTESIAN_POINT('Ctrl Pts',(-2.51566539374153,49.9965492175946,0.112583302491982));
#13900=CARTESIAN_POINT('Ctrl Pts',(-2.51343913234902,50.0006110695374,0.387416697508021));
#13901=CARTESIAN_POINT('Ctrl Pts',(-2.51262481849839,49.5480601771088,0.415916747158344));
#13902=CARTESIAN_POINT('Ctrl Pts',(-2.39612581621068,49.0950781816461,0.444416796808667));
#13903=CARTESIAN_POINT('Ctrl Pts',(-2.16649440645853,48.7095058462719,0.472916846458989));
#13904=CARTESIAN_POINT('Ctrl Pts',(-1.74003948947585,47.9934486725154,0.525845086200883));
#13905=CARTESIAN_POINT('Ctrl Pts',(-0.923399457867387,47.509882316713,0.578773325942776));
#13906=CARTESIAN_POINT('Ctrl Pts',(-0.0905132172451013,47.4799853381815,
0.63170156568467));
#13907=CARTESIAN_POINT('Ctrl Pts',(0.742373023377197,47.45008835965,0.684629805426564));
#13908=CARTESIAN_POINT('Ctrl Pts',(1.59150547301333,47.8738607583895,0.73755804516846));
#13909=CARTESIAN_POINT('Ctrl Pts',(2.06826581498737,48.5574101224076,0.790486284910355));
#13910=CARTESIAN_POINT('Ctrl Pts',(2.54502615696142,49.2409594864258,0.84341452465225));
#13911=CARTESIAN_POINT('Ctrl Pts',(2.64941439127338,50.1842858157225,0.896342764394143));
#13912=CARTESIAN_POINT('Ctrl Pts',(2.33361478103381,50.95554584747,0.949271004136037));
#13913=CARTESIAN_POINT('Ctrl Pts',(2.01781517079425,51.7268058792174,1.00219924387793));
#13914=CARTESIAN_POINT('Ctrl Pts',(1.28182771600316,52.3259996134155,1.05512748361983));
#13915=CARTESIAN_POINT('Ctrl Pts',(0.462561219916565,52.4788730216424,1.10805572336172));
#13916=CARTESIAN_POINT('Ctrl Pts',(-0.356705276170035,52.6317464298693,
1.16098396310362));
#13917=CARTESIAN_POINT('Ctrl Pts',(-1.25925081355216,52.338299512125,1.21391220284551));
#13918=CARTESIAN_POINT('Ctrl Pts',(-1.83195103174541,51.7328440723438,1.26684044258741));
#13919=CARTESIAN_POINT('Ctrl Pts',(-2.26684204543177,51.2730797461156,1.30703252756094));
#13920=CARTESIAN_POINT('Ctrl Pts',(-2.51153043874408,50.6333982435079,1.34722461253448));
#13921=CARTESIAN_POINT('Ctrl Pts',(-2.51733703324273,49.9976965409071,1.38741669750802));
#13922=CARTESIAN_POINT('Origin',(0.,50.,5.));
#13923=CARTESIAN_POINT('',(-2.52130183071094,50.0008653446746,2.38741669750802));
#13924=CARTESIAN_POINT('',(-2.51579666705823,50.0021291253541,2.11258330249198));
#13925=CARTESIAN_POINT('',(-2.5175,50.,5.));
#13926=CARTESIAN_POINT('Ctrl Pts',(-2.51579666705823,50.0021291253541,2.11258330249198));
#13927=CARTESIAN_POINT('Ctrl Pts',(-2.51784694340528,50.257604699766,2.09645598497262));
#13928=CARTESIAN_POINT('Ctrl Pts',(-2.48205558212342,50.5125192663648,2.08032866745325));
#13929=CARTESIAN_POINT('Ctrl Pts',(-2.40604315257227,50.7548157476474,2.06420134993389));
#13930=CARTESIAN_POINT('Ctrl Pts',(-2.15657797711353,51.5500085151083,2.011273110192));
#13931=CARTESIAN_POINT('Ctrl Pts',(-1.47389705953297,52.2092935747538,1.9583448704501));
#13932=CARTESIAN_POINT('Ctrl Pts',(-0.67049187024376,52.4308904409638,1.9054166307082));
#13933=CARTESIAN_POINT('Ctrl Pts',(0.132913319045451,52.6524873071738,1.85248839096631));
#13934=CARTESIAN_POINT('Ctrl Pts',(1.05704278004332,52.4363959799482,1.79956015122442));
#13935=CARTESIAN_POINT('Ctrl Pts',(1.67888372485688,51.8815269103202,1.74663191148252));
#13936=CARTESIAN_POINT('Ctrl Pts',(2.30072466967044,51.3266578406921,1.69370367174063));
#13937=CARTESIAN_POINT('Ctrl Pts',(2.62027709829971,50.4330110286616,1.64077543199873));
#13938=CARTESIAN_POINT('Ctrl Pts',(2.49126884240055,49.6096529788875,1.58784719225684));
#13939=CARTESIAN_POINT('Ctrl Pts',(2.36226058650139,48.7862949291135,1.53491895251495));
#13940=CARTESIAN_POINT('Ctrl Pts',(1.7846916460738,48.0332256415959,1.48199071277305));
#13941=CARTESIAN_POINT('Ctrl Pts',(1.02293880729862,47.6951424070907,1.42906247303116));
#13942=CARTESIAN_POINT('Ctrl Pts',(0.261185968523444,47.3570591725854,1.37613423328926));
#13943=CARTESIAN_POINT('Ctrl Pts',(-0.684750768599321,47.4339619910925,
1.32320599354737));
#13944=CARTESIAN_POINT('Ctrl Pts',(-1.38187543823614,47.8906768280442,1.27027775380547));
#13945=CARTESIAN_POINT('Ctrl Pts',(-2.07421342145999,48.3442557112708,1.21771293670098));
#13946=CARTESIAN_POINT('Ctrl Pts',(-2.52114445696114,49.1724486921844,1.16514811959648));
#13947=CARTESIAN_POINT('Ctrl Pts',(-2.52165773822405,50.0001226503677,1.11258330249199));
#13948=CARTESIAN_POINT('Ctrl Pts',(-2.51733703324273,49.9976965409071,1.38741669750802));
#13949=CARTESIAN_POINT('Ctrl Pts',(-2.51917703945939,49.7962540112111,1.40015285227638));
#13950=CARTESIAN_POINT('Ctrl Pts',(-2.49702989601834,49.5952111103643,1.41288900704473));
#13951=CARTESIAN_POINT('Ctrl Pts',(-2.44934665571188,49.4004193485444,1.42562516181309));
#13952=CARTESIAN_POINT('Ctrl Pts',(-2.25118716248072,48.5909140263443,1.47855340155498));
#13953=CARTESIAN_POINT('Ctrl Pts',(-1.61201327701402,47.8893673437622,1.53148164129688));
#13954=CARTESIAN_POINT('Ctrl Pts',(-0.824403714088269,47.6169036636344,
1.58440988103877));
#13955=CARTESIAN_POINT('Ctrl Pts',(-0.0367941511625192,47.3444399835067,
1.63733812078066));
#13956=CARTESIAN_POINT('Ctrl Pts',(0.899251089222284,47.5010593058334,1.69026636052256));
#13957=CARTESIAN_POINT('Ctrl Pts',(1.55526611555618,48.0150718634765,1.74319460026445));
#13958=CARTESIAN_POINT('Ctrl Pts',(2.21128114189008,48.5290844211196,1.79612284000635));
#13959=CARTESIAN_POINT('Ctrl Pts',(2.58726595417309,49.4004902140791,1.84905107974824));
#13960=CARTESIAN_POINT('Ctrl Pts',(2.5111160610797,50.230409713109,1.90197931949014));
#13961=CARTESIAN_POINT('Ctrl Pts',(2.43496616798631,51.0603292121388,1.95490755923203));
#13962=CARTESIAN_POINT('Ctrl Pts',(1.90668156951655,51.8487624172389,2.00783579897393));
#13963=CARTESIAN_POINT('Ctrl Pts',(1.16808045474115,52.2348109074211,2.06076403871582));
#13964=CARTESIAN_POINT('Ctrl Pts',(0.429479339965766,52.6208593976033,2.11369227845772));
#13965=CARTESIAN_POINT('Ctrl Pts',(-0.519438291115244,52.6045231728675,
2.16662051819961));
#13966=CARTESIAN_POINT('Ctrl Pts',(-1.24431337085575,52.1932798198687,2.21954875794151));
#13967=CARTESIAN_POINT('Ctrl Pts',(-1.96918845059626,51.78203646687,2.2724769976834));
#13968=CARTESIAN_POINT('Ctrl Pts',(-2.47002097899627,50.9758859856083,2.32540523742529));
#13969=CARTESIAN_POINT('Ctrl Pts',(-2.51755893192147,50.1438371940777,2.37833347716719));
#13970=CARTESIAN_POINT('Ctrl Pts',(-2.52027832269835,50.0962401548622,2.3813612172808));
#13971=CARTESIAN_POINT('Ctrl Pts',(-2.52151436629643,50.0485583668156,2.38438895739441));
#13972=CARTESIAN_POINT('Ctrl Pts',(-2.52130183071094,50.0008653446746,2.38741669750802));
#13973=CARTESIAN_POINT('Origin',(0.,50.,5.));
#13974=CARTESIAN_POINT('',(-2.51477537127748,50.0017637133429,3.38741669750802));
#13975=CARTESIAN_POINT('',(-2.51410548455075,49.9986698388504,3.11258330249199));
#13976=CARTESIAN_POINT('',(-2.5175,50.,5.));
#13977=CARTESIAN_POINT('Ctrl Pts',(-2.51410548455075,49.9986698388504,3.11258330249199));
#13978=CARTESIAN_POINT('Ctrl Pts',(-2.5116808105572,50.5047191991178,3.08069209009065));
#13979=CARTESIAN_POINT('Ctrl Pts',(-2.36361132718456,51.0120740142689,3.04880087768932));
#13980=CARTESIAN_POINT('Ctrl Pts',(-2.07960156886363,51.4262003567888,3.01690966528799));
#13981=CARTESIAN_POINT('Ctrl Pts',(-1.60824487071502,52.1135049993496,2.9639814255461));
#13982=CARTESIAN_POINT('Ctrl Pts',(-0.762449251371702,52.5440176887533,
2.9110531858042));
#13983=CARTESIAN_POINT('Ctrl Pts',(0.0706293316935971,52.5206748274805,
2.85812494606231));
#13984=CARTESIAN_POINT('Ctrl Pts',(0.90370791475889,52.4973319662077,2.80519670632041));
#13985=CARTESIAN_POINT('Ctrl Pts',(1.72406946154617,52.0201335542584,2.75226846657852));
#13986=CARTESIAN_POINT('Ctrl Pts',(2.15620024718853,51.3075131635299,2.69934022683662));
#13987=CARTESIAN_POINT('Ctrl Pts',(2.5883310328309,50.5948927728014,2.64641198709473));
#13988=CARTESIAN_POINT('Ctrl Pts',(2.63223105732835,49.6468504032936,2.59348374735283));
#13989=CARTESIAN_POINT('Ctrl Pts',(2.26780545235797,48.8973447372696,2.54055550761094));
#13990=CARTESIAN_POINT('Ctrl Pts',(1.90337984738758,48.1478390712456,2.48762726786904));
#13991=CARTESIAN_POINT('Ctrl Pts',(1.13062861294936,47.5968701087052,2.43469902812715));
#13992=CARTESIAN_POINT('Ctrl Pts',(0.303272233527588,47.4966391080133,2.38177078838526));
#13993=CARTESIAN_POINT('Ctrl Pts',(-0.524084145894187,47.3964081073213,
2.32884254864336));
#13994=CARTESIAN_POINT('Ctrl Pts',(-1.40604567029951,47.7469150684777,2.27591430890147));
#13995=CARTESIAN_POINT('Ctrl Pts',(-1.93890171583371,48.387718786694,2.22298606915957));
#13996=CARTESIAN_POINT('Ctrl Pts',(-2.30939568999827,48.8332686086602,2.18618514693704));
#13997=CARTESIAN_POINT('Ctrl Pts',(-2.51111814192273,49.4191594695261,2.14938422471451));
#13998=CARTESIAN_POINT('Ctrl Pts',(-2.51579666705823,50.0021291253541,2.11258330249198));
#13999=CARTESIAN_POINT('Ctrl Pts',(-2.52130183071094,50.0008653446746,2.38741669750802));
#14000=CARTESIAN_POINT('Ctrl Pts',(-2.5177990096276,49.2148316877844,2.43731719713631));
#14001=CARTESIAN_POINT('Ctrl Pts',(-2.12082327730247,48.4257465499517,2.48721769676459));
#14002=CARTESIAN_POINT('Ctrl Pts',(-1.48602084271957,47.9627140408783,2.53711819639287));
#14003=CARTESIAN_POINT('Ctrl Pts',(-0.812701423142097,47.4715867810093,
2.59004643613477));
#14004=CARTESIAN_POINT('Ctrl Pts',(0.128180793463234,47.347279363071,2.64297467587666));
#14005=CARTESIAN_POINT('Ctrl Pts',(0.905944761878115,47.6466925048363,2.69590291561856));
#14006=CARTESIAN_POINT('Ctrl Pts',(1.683708730293,47.9461056466016,2.74883115536045));
#14007=CARTESIAN_POINT('Ctrl Pts',(2.29835445051743,48.6692393480704,2.80175939510235));
#14008=CARTESIAN_POINT('Ctrl Pts',(2.46853291167733,49.4850851180826,2.85468763484424));
#14009=CARTESIAN_POINT('Ctrl Pts',(2.63871137283723,50.3009308880947,2.90761587458614));
#14010=CARTESIAN_POINT('Ctrl Pts',(2.36442257493259,51.2094887266502,2.96054411432803));
#14011=CARTESIAN_POINT('Ctrl Pts',(1.77121995432369,51.7948737935868,3.01347235406992));
#14012=CARTESIAN_POINT('Ctrl Pts',(1.17801733371478,52.3802588605235,3.06640059381182));
#14013=CARTESIAN_POINT('Ctrl Pts',(0.265900890401605,52.6424711558412,3.11932883355372));
#14014=CARTESIAN_POINT('Ctrl Pts',(-0.547615609742164,52.461485164032,3.17225707329561));
#14015=CARTESIAN_POINT('Ctrl Pts',(-1.36113210988593,52.2804991722228,3.2251853130375));
#14016=CARTESIAN_POINT('Ctrl Pts',(-2.07604866686029,51.6563148932866,3.2781135527794));
#14017=CARTESIAN_POINT('Ctrl Pts',(-2.36511813044588,50.8746475269621,3.33104179252129));
#14018=CARTESIAN_POINT('Ctrl Pts',(-2.46774931324276,50.597124452181,3.34983342751687));
#14019=CARTESIAN_POINT('Ctrl Pts',(-2.51670106273314,50.2997501138417,3.36862506251244));
#14020=CARTESIAN_POINT('Ctrl Pts',(-2.51477537127748,50.0017637133429,3.38741669750802));
#14021=CARTESIAN_POINT('Origin',(0.,50.,5.));
#14022=CARTESIAN_POINT('',(-2.51492115541711,49.9981671707055,4.38741669750802));
#14023=CARTESIAN_POINT('',(-2.52064984019739,49.9985765242422,4.11258330249199));
#14024=CARTESIAN_POINT('',(-2.5175,50.,5.));
#14025=CARTESIAN_POINT('Ctrl Pts',(-2.52064984019739,49.9985765242422,4.11258330249199));
#14026=CARTESIAN_POINT('Ctrl Pts',(-2.51556776575615,50.7497542365495,4.06492819520869));
#14027=CARTESIAN_POINT('Ctrl Pts',(-2.15787617855472,51.5051323059894,4.01727308792539));
#14028=CARTESIAN_POINT('Ctrl Pts',(-1.57089146705521,51.9725846320086,3.96961798064209));
#14029=CARTESIAN_POINT('Ctrl Pts',(-0.918955729079003,52.4917614881716,
3.9166897409002));
#14030=CARTESIAN_POINT('Ctrl Pts',(0.0158240478079662,52.6557681645712,
3.8637615011583));
#14031=CARTESIAN_POINT('Ctrl Pts',(0.805560141658845,52.3895319602189,3.81083326141641));
#14032=CARTESIAN_POINT('Ctrl Pts',(1.59529623550971,52.1232957558667,3.75790502167451));
#14033=CARTESIAN_POINT('Ctrl Pts',(2.2399886463245,51.4268166707627,3.70497678193262));
#14034=CARTESIAN_POINT('Ctrl Pts',(2.44453474790488,50.6189022524807,3.65204854219073));
#14035=CARTESIAN_POINT('Ctrl Pts',(2.64908084948526,49.8109878341986,3.59912030244883));
#14036=CARTESIAN_POINT('Ctrl Pts',(2.41348064183123,48.8916380827385,3.54619206270694));
#14037=CARTESIAN_POINT('Ctrl Pts',(1.84557817412316,48.2816777553516,3.49326382296504));
#14038=CARTESIAN_POINT('Ctrl Pts',(1.27767570641509,47.6717174279646,3.44033558322315));
#14039=CARTESIAN_POINT('Ctrl Pts',(0.377470978652977,47.3711465246507,3.38740734348125));
#14040=CARTESIAN_POINT('Ctrl Pts',(-0.442974730529885,47.517548889903,3.33447910373936));
#14041=CARTESIAN_POINT('Ctrl Pts',(-1.26342043971276,47.6639512551553,3.28155086399746));
#14042=CARTESIAN_POINT('Ctrl Pts',(-2.00410713031638,48.2573268889739,3.22862262425557));
#14043=CARTESIAN_POINT('Ctrl Pts',(-2.32599158714125,49.0260630037421,3.17569438451367));
#14044=CARTESIAN_POINT('Ctrl Pts',(-2.4539288121793,49.3316073170032,3.15465735717311));
#14045=CARTESIAN_POINT('Ctrl Pts',(-2.51570491992036,49.6648545516281,3.13362032983255));
#14046=CARTESIAN_POINT('Ctrl Pts',(-2.51410548455075,49.9986698388504,3.11258330249199));
#14047=CARTESIAN_POINT('Ctrl Pts',(-2.51477537127748,50.0017637133429,3.38741669750802));
#14048=CARTESIAN_POINT('Ctrl Pts',(-2.51127718880957,49.4604460485417,3.42155330225434));
#14049=CARTESIAN_POINT('Ctrl Pts',(-2.33988439025294,48.917108589911,3.45568990700066));
#14050=CARTESIAN_POINT('Ctrl Pts',(-2.01739407194983,48.48708452822,3.48982651174697));
#14051=CARTESIAN_POINT('Ctrl Pts',(-1.51737817967137,47.8203393495149,3.54275475148887));
#14052=CARTESIAN_POINT('Ctrl Pts',(-0.654124024917635,47.4259994458174,
3.59568299123076));
#14053=CARTESIAN_POINT('Ctrl Pts',(0.177220933403488,47.4845706513577,3.64861123097266));
#14054=CARTESIAN_POINT('Ctrl Pts',(1.00856589172461,47.5431418568979,3.70153947071455));
#14055=CARTESIAN_POINT('Ctrl Pts',(1.80800165361312,48.0546241716759,3.75446771045645));
#14056=CARTESIAN_POINT('Ctrl Pts',(2.20959310192558,48.7848907905357,3.80739595019834));
#14057=CARTESIAN_POINT('Ctrl Pts',(2.61118455023805,49.5151574093954,3.86032418994024));
#14058=CARTESIAN_POINT('Ctrl Pts',(2.61493168497446,50.4642083323369,3.91325242968213));
#14059=CARTESIAN_POINT('Ctrl Pts',(2.2191192862364,51.1976233382602,3.96618066942402));
#14060=CARTESIAN_POINT('Ctrl Pts',(1.82330688749833,51.9310383441836,4.01910890916592));
#14061=CARTESIAN_POINT('Ctrl Pts',(1.02793495528578,52.4488174330888,4.07203714890781));
#14062=CARTESIAN_POINT('Ctrl Pts',(0.197078422081479,52.5139515036224,4.12496538864971));
#14063=CARTESIAN_POINT('Ctrl Pts',(-0.633778111122818,52.5790855741559,
4.1778936283916));
#14064=CARTESIAN_POINT('Ctrl Pts',(-1.50011924531886,52.1915746263178,4.2308218681335));
#14065=CARTESIAN_POINT('Ctrl Pts',(-2.00538448193382,51.5287985958244,4.28375010787539));
#14066=CARTESIAN_POINT('Ctrl Pts',(-2.33525957441895,51.0960886278467,4.31830563775293));
#14067=CARTESIAN_POINT('Ctrl Pts',(-2.51122754678017,50.5460480475906,4.35286116763048));
#14068=CARTESIAN_POINT('Ctrl Pts',(-2.51492115541711,49.9981671707055,4.38741669750802));
#14069=CARTESIAN_POINT('Origin',(0.,50.,5.));
#14070=CARTESIAN_POINT('',(-2.52139129543236,49.9992487982722,5.38741669750802));
#14071=CARTESIAN_POINT('',(-2.51841387510379,50.0022201728711,5.11258330249199));
#14072=CARTESIAN_POINT('',(-2.5175,50.,5.));
#14073=CARTESIAN_POINT('Ctrl Pts',(-2.51841387510379,50.0022201728711,5.11258330249199));
#14074=CARTESIAN_POINT('Ctrl Pts',(-2.51993725434446,50.167966042206,5.10209254006862));
#14075=CARTESIAN_POINT('Ctrl Pts',(-2.50497422321175,50.3334381998588,5.09160177764525));
#14076=CARTESIAN_POINT('Ctrl Pts',(-2.47252158136002,50.4954060568224,5.08111101522188));
#14077=CARTESIAN_POINT('Ctrl Pts',(-2.3087907542888,51.3125700738777,5.02818277547998));
#14078=CARTESIAN_POINT('Ctrl Pts',(-1.69987449903624,52.0405346440253,4.97525453573809));
#14079=CARTESIAN_POINT('Ctrl Pts',(-0.924499202043288,52.3460799979661,
4.92232629599619));
#14080=CARTESIAN_POINT('Ctrl Pts',(-0.149123905050339,52.651625351907,4.8693980562543));
#14081=CARTESIAN_POINT('Ctrl Pts',(0.792710433683001,52.5347514896411,4.8164698165124));
#14082=CARTESIAN_POINT('Ctrl Pts',(1.46988692476992,52.048956456299,4.76354157677051));
#14083=CARTESIAN_POINT('Ctrl Pts',(2.14706341585683,51.5631614229569,4.71061333702861));
#14084=CARTESIAN_POINT('Ctrl Pts',(2.55958205929732,50.7084452185386,4.65768509728672));
#14085=CARTESIAN_POINT('Ctrl Pts',(2.51861585329202,49.8760471259917,4.60475685754483));
#14086=CARTESIAN_POINT('Ctrl Pts',(2.47764964728673,49.0436490334448,4.55182861780293));
#14087=CARTESIAN_POINT('Ctrl Pts',(1.98319859183565,48.2335690527693,4.49890037806103));
#14088=CARTESIAN_POINT('Ctrl Pts',(1.26159357360843,47.8166146042215,4.44597213831914));
#14089=CARTESIAN_POINT('Ctrl Pts',(0.539988555381206,47.3996601556737,4.39304389857725));
#14090=CARTESIAN_POINT('Ctrl Pts',(-0.408770425622154,47.3758312392538,
4.34011565883535));
#14091=CARTESIAN_POINT('Ctrl Pts',(-1.1503967822133,47.7560353445703,4.28718741909346));
#14092=CARTESIAN_POINT('Ctrl Pts',(-1.89202313880445,48.1362394498869,4.23425917935156));
#14093=CARTESIAN_POINT('Ctrl Pts',(-2.42651687098339,48.9204765769399,4.18133093960967));
#14094=CARTESIAN_POINT('Ctrl Pts',(-2.50921788754013,49.7497686584296,4.12840269986777));
#14095=CARTESIAN_POINT('Ctrl Pts',(-2.51745722096386,49.832389335291,4.12312956740918));
#14096=CARTESIAN_POINT('Ctrl Pts',(-2.52121218184807,49.9154572154682,4.11785643495058));
#14097=CARTESIAN_POINT('Ctrl Pts',(-2.52064984019739,49.9985765242422,4.11258330249199));
#14098=CARTESIAN_POINT('Ctrl Pts',(-2.51492115541711,49.9981671707055,4.38741669750802));
#14099=CARTESIAN_POINT('Ctrl Pts',(-2.51688499738623,49.7068662869712,4.40578940737237));
#14100=CARTESIAN_POINT('Ctrl Pts',(-2.47014850145045,49.4161759310116,4.42416211723673));
#14101=CARTESIAN_POINT('Ctrl Pts',(-2.37195102004796,49.1440558280711,4.44253482710108));
#14102=CARTESIAN_POINT('Ctrl Pts',(-2.08906298251325,48.3601302039597,4.49546306684297));
#14103=CARTESIAN_POINT('Ctrl Pts',(-1.37909756840994,47.7303200688855,4.54839130658487));
#14104=CARTESIAN_POINT('Ctrl Pts',(-0.567035582013418,47.5429158102107,
4.60131954632676));
#14105=CARTESIAN_POINT('Ctrl Pts',(0.245026404383105,47.3555115515358,4.65424778606865));
#14106=CARTESIAN_POINT('Ctrl Pts',(1.15918496307284,47.6105131692602,4.70717602581055));
#14107=CARTESIAN_POINT('Ctrl Pts',(1.7569915643907,48.1911957790756,4.76010426555244));
#14108=CARTESIAN_POINT('Ctrl Pts',(2.35479816570856,48.771878388891,4.81303250529434));
#14109=CARTESIAN_POINT('Ctrl Pts',(2.63625280965454,49.6782419907974,4.86596074503623));
#14110=CARTESIAN_POINT('Ctrl Pts',(2.47252195766438,50.4954061322205,4.91888898477813));
#14111=CARTESIAN_POINT('Ctrl Pts',(2.30879110567422,51.3125702736437,4.97181722452002));
#14112=CARTESIAN_POINT('Ctrl Pts',(1.69987475774791,52.0405349545835,5.02474546426192));
#14113=CARTESIAN_POINT('Ctrl Pts',(0.924499342747056,52.3460803550268,5.07767370400381));
#14114=CARTESIAN_POINT('Ctrl Pts',(0.149123927746205,52.65162575547,5.13060194374571));
#14115=CARTESIAN_POINT('Ctrl Pts',(-0.792710554329193,52.5347518754165,
5.1835301834876));
#14116=CARTESIAN_POINT('Ctrl Pts',(-1.46988714847869,52.048956768139,5.23645842322949));
#14117=CARTESIAN_POINT('Ctrl Pts',(-2.11368593801667,51.5871063369063,5.286777847989));
#14118=CARTESIAN_POINT('Ctrl Pts',(-2.5182736560907,50.7918063994386,5.33709727274851));
#14119=CARTESIAN_POINT('Ctrl Pts',(-2.52139129543236,49.9992487982722,5.38741669750802));
#14120=CARTESIAN_POINT('Origin',(0.,50.,5.));
#14121=CARTESIAN_POINT('',(-2.51713805421624,50.0023011578997,6.38741669750802));
#14122=CARTESIAN_POINT('',(-2.51340291777706,50.0000546149131,6.11258330249199));
#14123=CARTESIAN_POINT('',(-2.5175,50.,5.));
#14124=CARTESIAN_POINT('Ctrl Pts',(-2.51340291777706,50.0000546149131,6.11258330249199));
#14125=CARTESIAN_POINT('Ctrl Pts',(-2.51348357000391,50.4169542413391,6.08632864518665));
#14126=CARTESIAN_POINT('Ctrl Pts',(-2.41545869747094,50.8338181852126,6.06007398788131));
#14127=CARTESIAN_POINT('Ctrl Pts',(-2.21911894849843,51.1976231559884,6.03381933057598));
#14128=CARTESIAN_POINT('Ctrl Pts',(-1.82330661000076,51.9310380502898,5.98089109083408));
#14129=CARTESIAN_POINT('Ctrl Pts',(-1.02793479883965,52.4488170603922,5.92796285109219));
#14130=CARTESIAN_POINT('Ctrl Pts',(-0.197078392087235,52.5139511210127,
5.87503461135029));
#14131=CARTESIAN_POINT('Ctrl Pts',(0.633778014665187,52.5790851816333,5.8221063716084));
#14132=CARTESIAN_POINT('Ctrl Pts',(1.50011901700892,52.191574292772,5.76917813186651));
#14133=CARTESIAN_POINT('Ctrl Pts',(2.00538417672529,51.5287983631495,5.71624989212461));
#14134=CARTESIAN_POINT('Ctrl Pts',(2.51064933644165,50.866022433527,5.66332165238272));
#14135=CARTESIAN_POINT('Ctrl Pts',(2.65483865353065,49.9279814631433,5.61039341264082));
#14136=CARTESIAN_POINT('Ctrl Pts',(2.37195065904994,49.1440559583411,5.55746517289893));
#14137=CARTESIAN_POINT('Ctrl Pts',(2.08906266456923,48.360130453539,5.50453693315704));
#14138=CARTESIAN_POINT('Ctrl Pts',(1.3790973585188,47.7303204143184,5.45160869341514));
#14139=CARTESIAN_POINT('Ctrl Pts',(0.567035495713689,47.5429161841654,5.39868045367324));
#14140=CARTESIAN_POINT('Ctrl Pts',(-0.245026367091423,47.3555119540124,
5.34575221393135));
#14141=CARTESIAN_POINT('Ctrl Pts',(-1.15918478665122,47.610513532927,5.29282397418945));
#14142=CARTESIAN_POINT('Ctrl Pts',(-1.75699129698618,48.1911960543657,5.23989573444756));
#14143=CARTESIAN_POINT('Ctrl Pts',(-2.23630820506625,48.6567830728078,5.19745825712904));
#14144=CARTESIAN_POINT('Ctrl Pts',(-2.5122514657989,49.3317411088454,5.15502077981051));
#14145=CARTESIAN_POINT('Ctrl Pts',(-2.51841387510379,50.0022201728711,5.11258330249199));
#14146=CARTESIAN_POINT('Ctrl Pts',(-2.52139129543236,49.9992487982722,5.38741669750802));
#14147=CARTESIAN_POINT('Ctrl Pts',(-2.521552929717,49.9581585800472,5.39002551249041));
#14148=CARTESIAN_POINT('Ctrl Pts',(-2.5206354473163,49.9170757329839,5.39263432747279));
#14149=CARTESIAN_POINT('Ctrl Pts',(-2.51861623661168,49.8760471071268,5.39524314245518));
#14150=CARTESIAN_POINT('Ctrl Pts',(-2.47765002437156,49.0436488878934,5.44817138219707));
#14151=CARTESIAN_POINT('Ctrl Pts',(-1.98319889366771,48.2335687839283,5.50109962193897));
#14152=CARTESIAN_POINT('Ctrl Pts',(-1.26159376561614,47.8166142719222,5.55402786168086));
#14153=CARTESIAN_POINT('Ctrl Pts',(-0.539988637564569,47.3996597599162,
5.60695610142275));
#14154=CARTESIAN_POINT('Ctrl Pts',(0.40877048783472,47.3758308398693,5.65988434116465));
#14155=CARTESIAN_POINT('Ctrl Pts',(1.15039695729739,47.7560350030509,5.71281258090654));
#14156=CARTESIAN_POINT('Ctrl Pts',(1.89202342676006,48.1362391662326,5.76574082064844));
#14157=CARTESIAN_POINT('Ctrl Pts',(2.42651724028611,48.9204764126428,5.81866906039033));
#14158=CARTESIAN_POINT('Ctrl Pts',(2.50921826942949,49.749768620346,5.87159730013223));
#14159=CARTESIAN_POINT('Ctrl Pts',(2.59191929857286,50.5790608280491,5.92452553987412));
#14160=CARTESIAN_POINT('Ctrl Pts',(2.22282754333358,51.4534079970451,5.97745377961602));
#14161=CARTESIAN_POINT('Ctrl Pts',(1.57089170613635,51.9725849322246,6.03038201935791));
#14162=CARTESIAN_POINT('Ctrl Pts',(0.918955868939124,52.4917618674041,6.08331025909981));
#14163=CARTESIAN_POINT('Ctrl Pts',(-0.0158240502160405,52.655768568767,
6.1362384988417));
#14164=CARTESIAN_POINT('Ctrl Pts',(-0.805560264260574,52.389532323894,6.18916673858359));
#14165=CARTESIAN_POINT('Ctrl Pts',(-1.59529647830511,52.1232960790209,6.24209497832549));
#14166=CARTESIAN_POINT('Ctrl Pts',(-2.23998898723901,51.4268168879119,6.29502321806738));
#14167=CARTESIAN_POINT('Ctrl Pts',(-2.44453511994999,50.6189023466718,6.34795145780928));
#14168=CARTESIAN_POINT('Ctrl Pts',(-2.49537415657931,50.418098760649,6.36110653770886));
#14169=CARTESIAN_POINT('Ctrl Pts',(-2.51902319308404,50.2104112665728,6.37426161760844));
#14170=CARTESIAN_POINT('Ctrl Pts',(-2.51713805421624,50.0023011578997,6.38741669750802));
#14171=CARTESIAN_POINT('Origin',(0.,50.,5.));
#14172=CARTESIAN_POINT('',(-2.51354891404356,49.9993677900347,7.38741669750802));
#14173=CARTESIAN_POINT('',(-2.51821333355664,49.9977519369613,7.11258330249199));
#14174=CARTESIAN_POINT('',(-2.5175,50.,5.));
#14175=CARTESIAN_POINT('Ctrl Pts',(-2.51821333355664,49.9977519369613,7.11258330249199));
#14176=CARTESIAN_POINT('Ctrl Pts',(-2.51208745167034,50.6617483076158,7.07056475030469));
#14177=CARTESIAN_POINT('Ctrl Pts',(-2.24214997829159,51.3301494078962,7.02854619811738));
#14178=CARTESIAN_POINT('Ctrl Pts',(-1.77121968474941,51.7948735204092,6.98652764593008));
#14179=CARTESIAN_POINT('Ctrl Pts',(-1.17801715441916,52.3802584982467,6.93359940618819));
#14180=CARTESIAN_POINT('Ctrl Pts',(-0.265900849933291,52.642470753672,6.88067116644629));
#14181=CARTESIAN_POINT('Ctrl Pts',(0.547615526395802,52.4614847894114,6.8277429267044));
#14182=CARTESIAN_POINT('Ctrl Pts',(1.36113190272489,52.2804988251508,6.7748146869625));
#14183=CARTESIAN_POINT('Ctrl Pts',(2.07604835089721,51.6563146412042,6.72188644722061));
#14184=CARTESIAN_POINT('Ctrl Pts',(2.36511777048901,50.8746473938434,6.66895820747871));
#14185=CARTESIAN_POINT('Ctrl Pts',(2.65418719008082,50.0929801464827,6.61602996773682));
#14186=CARTESIAN_POINT('Ctrl Pts',(2.51740958109211,49.1538298357076,6.56310172799492));
#14187=CARTESIAN_POINT('Ctrl Pts',(2.01739376491279,48.4870847584785,6.51017348825303));
#14188=CARTESIAN_POINT('Ctrl Pts',(1.51737794873347,47.8203396812494,6.45724524851113));
#14189=CARTESIAN_POINT('Ctrl Pts',(0.654123925363523,47.4259998375662,6.40431700876924));
#14190=CARTESIAN_POINT('Ctrl Pts',(-0.177220906431141,47.4845710341917,
6.35138876902734));
#14191=CARTESIAN_POINT('Ctrl Pts',(-1.00856573822581,47.5431422308173,6.29846052928545));
#14192=CARTESIAN_POINT('Ctrl Pts',(-1.80800137844519,48.0546244677515,6.24553228954355));
#14193=CARTESIAN_POINT('Ctrl Pts',(-2.20959276563777,48.784890975469,6.19260404980166));
#14194=CARTESIAN_POINT('Ctrl Pts',(-2.41197774999261,49.1529142460188,6.1659304673651));
#14195=CARTESIAN_POINT('Ctrl Pts',(-2.51332097864539,49.5765028456433,6.13925688492854));
#14196=CARTESIAN_POINT('Ctrl Pts',(-2.51340291777706,50.0000546149131,6.11258330249199));
#14197=CARTESIAN_POINT('Ctrl Pts',(-2.51713805421624,50.0023011578997,6.38741669750802));
#14198=CARTESIAN_POINT('Ctrl Pts',(-2.51143851228367,49.3730996114068,6.42718985735034));
#14199=CARTESIAN_POINT('Ctrl Pts',(-2.27233134100759,48.7400349493151,6.46696301719265));
#14200=CARTESIAN_POINT('Ctrl Pts',(-1.84557845500972,48.2816774938369,6.50673617703496));
#14201=CARTESIAN_POINT('Ctrl Pts',(-1.27767590087041,47.6717170736132,6.55966441677686));
#14202=CARTESIAN_POINT('Ctrl Pts',(-0.377471036103719,47.3711461245372,
6.61259265651875));
#14203=CARTESIAN_POINT('Ctrl Pts',(0.442974797947392,47.5175485120787,6.66552089626065));
#14204=CARTESIAN_POINT('Ctrl Pts',(1.2634206319985,47.6639508996202,6.71844913600254));
#14205=CARTESIAN_POINT('Ctrl Pts',(2.00410743533403,48.2573266237792,6.77137737574443));
#14206=CARTESIAN_POINT('Ctrl Pts',(2.32599194114623,49.0260628555307,6.82430561548633));
#14207=CARTESIAN_POINT('Ctrl Pts',(2.64787644695843,49.7947990872822,6.87723385522822));
#14208=CARTESIAN_POINT('Ctrl Pts',(2.55095865524729,50.7388958266262,6.93016209497012));
#14209=CARTESIAN_POINT('Ctrl Pts',(2.07960188536427,51.4262005738175,6.98309033471202));
#14210=CARTESIAN_POINT('Ctrl Pts',(1.60824511548125,52.1135053210088,7.03601857445391));
#14211=CARTESIAN_POINT('Ctrl Pts',(0.762449367426351,52.5440180760474,7.0889468141958));
#14212=CARTESIAN_POINT('Ctrl Pts',(-0.0706293424360422,52.5206752111724,
7.14187505393769));
#14213=CARTESIAN_POINT('Ctrl Pts',(-0.903708052298439,52.4973323462974,
7.19480329367959));
#14214=CARTESIAN_POINT('Ctrl Pts',(-1.72406972396833,52.0201338615088,7.24773153342148));
#14215=CARTESIAN_POINT('Ctrl Pts',(-2.15620057536443,51.3075133624157,7.30065977316338));
#14216=CARTESIAN_POINT('Ctrl Pts',(-2.39230858225818,50.9181511931355,7.32957874794493));
#14217=CARTESIAN_POINT('Ctrl Pts',(-2.512517267736,50.4585080201858,7.35849772272647));
#14218=CARTESIAN_POINT('Ctrl Pts',(-2.51354891404356,49.9993677900347,7.38741669750802));
#14219=CARTESIAN_POINT('Origin',(0.,50.,5.));
#14220=CARTESIAN_POINT('',(-2.51945660451951,49.9980217824357,8.38741669750802));
#14221=CARTESIAN_POINT('',(-2.52079116141582,50.0013273547755,8.11258330249199));
#14222=CARTESIAN_POINT('',(-2.5175,50.,5.));
#14223=CARTESIAN_POINT('Ctrl Pts',(-2.52079116141582,50.0013273547755,8.11258330249199));
#14224=CARTESIAN_POINT('Ctrl Pts',(-2.52128051842586,50.0778319453862,8.10772909516462));
#14225=CARTESIAN_POINT('Ctrl Pts',(-2.51809961281036,50.1542952883015,8.10287488783724));
#14226=CARTESIAN_POINT('Ctrl Pts',(-2.51111567921584,50.2304096787005,8.09802068050987));
#14227=CARTESIAN_POINT('Ctrl Pts',(-2.43496579794733,51.0603290519682,8.04509244076797));
#14228=CARTESIAN_POINT('Ctrl Pts',(-1.90668127928963,51.8487621358105,7.99216420102608));
#14229=CARTESIAN_POINT('Ctrl Pts',(-1.16808027679305,52.234810566944,7.93923596128418));
#14230=CARTESIAN_POINT('Ctrl Pts',(-0.429479274296469,52.6208589980775,
7.88630772154228));
#14231=CARTESIAN_POINT('Ctrl Pts',(0.519438212038995,52.6045227765023,7.83337948180039));
#14232=CARTESIAN_POINT('Ctrl Pts',(1.24431318138389,52.1932794862502,7.7804512420585));
#14233=CARTESIAN_POINT('Ctrl Pts',(1.96918815072878,51.782036195998,7.7275230023166));
#14234=CARTESIAN_POINT('Ctrl Pts',(2.47002060308309,50.975885837069,7.67459476257471));
#14235=CARTESIAN_POINT('Ctrl Pts',(2.51755854881386,50.1438371720874,7.62166652283282));
#14236=CARTESIAN_POINT('Ctrl Pts',(2.56509649454462,49.3117885071058,7.56873828309093));
#14237=CARTESIAN_POINT('Ctrl Pts',(2.15933993365185,48.4538415360717,7.51581004334903));
#14238=CARTESIAN_POINT('Ctrl Pts',(1.48602061652768,47.9627143509944,7.46288180360713));
#14239=CARTESIAN_POINT('Ctrl Pts',(0.812701299403498,47.4715871659172,7.40995356386523));
#14240=CARTESIAN_POINT('Ctrl Pts',(-0.128180773952088,47.3472797667968,
7.35702532412334));
#14241=CARTESIAN_POINT('Ctrl Pts',(-0.90594462398342,47.6466928629692,7.30409708438145));
#14242=CARTESIAN_POINT('Ctrl Pts',(-1.68370847401475,47.9461059591416,7.25116884463955));
#14243=CARTESIAN_POINT('Ctrl Pts',(-2.29835410072182,48.6692395506069,7.19824060489766));
#14244=CARTESIAN_POINT('Ctrl Pts',(-2.46853253598805,49.4850851964644,7.14531236515576));
#14245=CARTESIAN_POINT('Ctrl Pts',(-2.50361009697133,49.6532491318698,7.13440267760117));
#14246=CARTESIAN_POINT('Ctrl Pts',(-2.5198038561686,49.8253520668056,7.12349299004658));
#14247=CARTESIAN_POINT('Ctrl Pts',(-2.51821333355664,49.9977519369613,7.11258330249199));
#14248=CARTESIAN_POINT('Ctrl Pts',(-2.51354891404356,49.9993677900347,7.38741669750802));
#14249=CARTESIAN_POINT('Ctrl Pts',(-2.51440541292469,49.6181779476241,7.41142596246837));
#14250=CARTESIAN_POINT('Ctrl Pts',(-2.4331162684414,49.2373347706455,7.43543522742872));
#14251=CARTESIAN_POINT('Ctrl Pts',(-2.26780579747753,48.8973445696587,7.45944449238906));
#14252=CARTESIAN_POINT('Ctrl Pts',(-1.9033801370722,48.1478387893924,7.51237273213096));
#14253=CARTESIAN_POINT('Ctrl Pts',(-1.13062878513921,47.5968697422575,7.56530097187285));
#14254=CARTESIAN_POINT('Ctrl Pts',(-0.303272279740653,47.4966387266282,
7.61822921161475));
#14255=CARTESIAN_POINT('Ctrl Pts',(0.524084225657901,47.3964077109989,7.67115745135664));
#14256=CARTESIAN_POINT('Ctrl Pts',(1.40604588452202,47.7469147268753,7.72408569109854));
#14257=CARTESIAN_POINT('Ctrl Pts',(1.93890201103807,48.3877185420343,7.77701393084044));
#14258=CARTESIAN_POINT('Ctrl Pts',(2.47175813755411,49.0285223571934,7.82994217058233));
#14259=CARTESIAN_POINT('Ctrl Pts',(2.6555087317221,49.9596229716351,7.88287041032422));
#14260=CARTESIAN_POINT('Ctrl Pts',(2.40604351852937,50.7548158611892,7.93579865006612));
#14261=CARTESIAN_POINT('Ctrl Pts',(2.15657830533664,51.5500087507433,7.98872688980801));
#14262=CARTESIAN_POINT('Ctrl Pts',(1.4738972847832,52.2092939154097,8.0416551295499));
#14263=CARTESIAN_POINT('Ctrl Pts',(0.670491972751082,52.4308908134011,8.09458336929179));
#14264=CARTESIAN_POINT('Ctrl Pts',(-0.132913339281037,52.6524877113925,
8.14751160903369));
#14265=CARTESIAN_POINT('Ctrl Pts',(-1.05704294279184,52.4363963427089,8.20043984877559));
#14266=CARTESIAN_POINT('Ctrl Pts',(-1.67888398130339,51.881527192142,8.25336808851749));
#14267=CARTESIAN_POINT('Ctrl Pts',(-2.20385216862142,51.4130977477473,8.298050958181));
#14268=CARTESIAN_POINT('Ctrl Pts',(-2.51337907056068,50.7032211259283,8.34273382784451));
#14269=CARTESIAN_POINT('Ctrl Pts',(-2.51945660451951,49.9980217824357,8.38741669750802));
#14270=CARTESIAN_POINT('Origin',(0.,50.,5.));
#14271=CARTESIAN_POINT('',(-2.51977158007336,50.0018123497868,9.38741669750802));
#14272=CARTESIAN_POINT('',(-2.51421069693398,50.0014124180709,9.11258330249199));
#14273=CARTESIAN_POINT('',(-2.5175,50.,5.));
#14274=CARTESIAN_POINT('',(1.91346599666507,51.6359872033749,10.));
#14275=CARTESIAN_POINT('Ctrl Pts',(-2.51977158007336,50.0018123497868,9.38741669750802));
#14276=CARTESIAN_POINT('Ctrl Pts',(-2.51384336591692,49.2855430820957,9.43282641244633));
#14277=CARTESIAN_POINT('Ctrl Pts',(-2.19294820505509,48.5647754397593,9.47823612738464));
#14278=CARTESIAN_POINT('Ctrl Pts',(-1.65296056616486,48.0958821170945,9.52364584232295));
#14279=CARTESIAN_POINT('Ctrl Pts',(-1.02356671844595,47.5493537315036,9.57657408206485));
#14280=CARTESIAN_POINT('Ctrl Pts',(-0.0965236035471523,47.3450105607878,
9.62950232180674));
#14281=CARTESIAN_POINT('Ctrl Pts',(0.703763603554138,47.5780839006293,9.68243056154863));
#14282=CARTESIAN_POINT('Ctrl Pts',(1.50405081065543,47.8111572404708,9.73535880129053));
#14283=CARTESIAN_POINT('Ctrl Pts',(2.17758210995922,48.4816470908697,9.78828704103243));
#14284=CARTESIAN_POINT('Ctrl Pts',(2.41595103931381,49.2787700048902,9.84121528077432));
#14285=CARTESIAN_POINT('Ctrl Pts',(2.6543199686684,50.0758929189107,9.89414352051622));
#14286=CARTESIAN_POINT('Ctrl Pts',(2.45752652807378,50.9996488965529,9.94707176025811));
#14287=CARTESIAN_POINT('Ctrl Pts',(1.91346599666507,51.6359872033749,10.));
#14288=CARTESIAN_POINT('',(-1.91709562399829,51.6387694827081,10.));
#14289=CARTESIAN_POINT('Origin',(0.,50.,10.));
#14290=CARTESIAN_POINT('Ctrl Pts',(-1.91709820558801,51.6387714616175,10.));
#14291=CARTESIAN_POINT('Ctrl Pts',(-1.38628658638899,52.2578908816981,9.94821753066413));
#14292=CARTESIAN_POINT('Ctrl Pts',(-0.526694367197532,52.597340211881,9.89643506132826));
#14293=CARTESIAN_POINT('Ctrl Pts',(0.283636601049879,52.5054918828108,9.84465259199238));
#14294=CARTESIAN_POINT('Ctrl Pts',(1.11189744507203,52.4116112617576,9.79172435225049));
#14295=CARTESIAN_POINT('Ctrl Pts',(1.88869295170318,51.8671355152453,9.73879611250859));
#14296=CARTESIAN_POINT('Ctrl Pts',(2.2589558309103,51.1206234649951,9.6858678727667));
#14297=CARTESIAN_POINT('Ctrl Pts',(2.62921871011742,50.374111414745,9.6329396330248));
#14298=CARTESIAN_POINT('Ctrl Pts',(2.59294896190052,49.425563060757,9.58001139328291));
#14299=CARTESIAN_POINT('Ctrl Pts',(2.16649410945695,48.7095058870182,9.52708315354102));
#14300=CARTESIAN_POINT('Ctrl Pts',(1.74003925701338,47.9934487132793,9.47415491379912));
#14301=CARTESIAN_POINT('Ctrl Pts',(0.923399300343145,47.5098827197895,9.42122667405723));
#14302=CARTESIAN_POINT('Ctrl Pts',(0.0905131805637632,47.4799858088808,
9.36829843431533));
#14303=CARTESIAN_POINT('Ctrl Pts',(-0.742372939215617,47.4500888979721,
9.31537019457344));
#14304=CARTESIAN_POINT('Ctrl Pts',(-1.59150522210415,47.8738610696445,9.26244195483154));
#14305=CARTESIAN_POINT('Ctrl Pts',(-2.06826548542263,48.5574102936455,9.20951371508965));
#14306=CARTESIAN_POINT('Ctrl Pts',(-2.35930463112246,48.9746841260163,9.1772035775571));
#14307=CARTESIAN_POINT('Ctrl Pts',(-2.51157883686813,49.4887642305379,9.14489344002454));
#14308=CARTESIAN_POINT('Ctrl Pts',(-2.51421069693398,50.0014124180709,9.11258330249199));
#14309=CARTESIAN_POINT('Origin',(0.,50.,12.2084234471775));
#14310=CARTESIAN_POINT('',(-3.07857599143262,50.0001497381948,0.791576552822544));
#14311=CARTESIAN_POINT('',(-3.06854227339611,50.0007460267024,0.708423447177453));
#14312=CARTESIAN_POINT('',(-3.0735,50.0000000000001,12.2084234471775));
#14313=CARTESIAN_POINT('',(0.793799282532843,47.0307770462543,0.));
#14314=CARTESIAN_POINT('Ctrl Pts',(-3.06854227339611,50.0007460267024,0.708423447177453));
#14315=CARTESIAN_POINT('Ctrl Pts',(-3.06939439432918,50.4743080180887,0.683995257085881));
#14316=CARTESIAN_POINT('Ctrl Pts',(-2.74351660027806,51.9727061273031,0.606638827252413));
#14317=CARTESIAN_POINT('Ctrl Pts',(-0.409110687221481,53.6089533032289,
0.47635415767705));
#14318=CARTESIAN_POINT('Ctrl Pts',(2.81294218225317,52.3024584702958,0.317569438451368));
#14319=CARTESIAN_POINT('Ctrl Pts',(3.45486176146768,48.8813761711215,0.158784719225683));
#14320=CARTESIAN_POINT('Ctrl Pts',(1.78123794632758,47.2947612990625,0.0529282397418946));
#14321=CARTESIAN_POINT('Ctrl Pts',(0.793799282532844,47.0307770462543,0.));
#14322=CARTESIAN_POINT('',(-0.793799282532893,47.0307770462543,0.));
#14323=CARTESIAN_POINT('Origin',(0.,50.,0.));
#14324=CARTESIAN_POINT('Ctrl Pts',(-3.07857599143262,50.0001497381948,0.791576552822544));
#14325=CARTESIAN_POINT('Ctrl Pts',(-3.07858032390664,50.0071359194187,0.791213130185147));
#14326=CARTESIAN_POINT('Ctrl Pts',(-3.07539543013204,51.0315729209784,0.737921467805856));
#14327=CARTESIAN_POINT('Ctrl Pts',(-1.94901659367837,53.0656756689436,0.631701565684669));
#14328=CARTESIAN_POINT('Ctrl Pts',(1.51908697082356,53.300340014212,0.472916846458987));
#14329=CARTESIAN_POINT('Ctrl Pts',(3.59644503276003,50.5125594541255,0.314132127233302));
#14330=CARTESIAN_POINT('Ctrl Pts',(2.3901758303772,47.2810813042181,0.15649317841364));
#14331=CARTESIAN_POINT('Ctrl Pts',(0.166672989744518,46.7696415803318,0.051782469335873));
#14332=CARTESIAN_POINT('Ctrl Pts',(-0.795528245027205,47.0254639548254,
-4.66206934168767E-17));
#14333=CARTESIAN_POINT('Origin',(0.,50.,12.2084234471775));
#14334=CARTESIAN_POINT('',(-3.0714204791275,50.0025993512516,1.79157655282254));
#14335=CARTESIAN_POINT('',(-3.07330104137895,49.9971878127024,1.70842344717745));
#14336=CARTESIAN_POINT('',(-3.0735,50.0000000000001,12.2084234471775));
#14337=CARTESIAN_POINT('Ctrl Pts',(-3.07330104137895,49.9971878127024,1.70842344717745));
#14338=CARTESIAN_POINT('Ctrl Pts',(-3.06621203713203,50.7732867930175,1.66823136220391));
#14339=CARTESIAN_POINT('Ctrl Pts',(-2.37409258821072,52.5826738386258,1.57511103748848));
#14340=CARTESIAN_POINT('Ctrl Pts',(0.666391278186825,53.5712340631145,1.42906247303115));
#14341=CARTESIAN_POINT('Ctrl Pts',(3.36199101081887,51.3766498223304,1.27027775380547));
#14342=CARTESIAN_POINT('Ctrl Pts',(2.97966262373907,47.9216585932218,1.11149303457979));
#14343=CARTESIAN_POINT('Ctrl Pts',(-0.130337674918302,46.3695658811752,
0.952708315354101));
#14344=CARTESIAN_POINT('Ctrl Pts',(-2.66118372910024,47.8681845578855,0.818351786219992));
#14345=CARTESIAN_POINT('Ctrl Pts',(-3.06754811505652,49.4482474495905,0.736923496827775));
#14346=CARTESIAN_POINT('Ctrl Pts',(-3.06854227339611,50.0007460267024,0.708423447177453));
#14347=CARTESIAN_POINT('Ctrl Pts',(-3.0714204791275,50.0025993512516,1.79157655282254));
#14348=CARTESIAN_POINT('Ctrl Pts',(-3.07392356725168,50.3144977337562,1.77544923530318));
#14349=CARTESIAN_POINT('Ctrl Pts',(-2.88682155748466,51.6470826375239,1.70639367804192));
#14350=CARTESIAN_POINT('Ctrl Pts',(-0.965959409052926,53.5021157627911,
1.58440988103877));
#14351=CARTESIAN_POINT('Ctrl Pts',(2.41872209844688,52.7106678650022,1.42562516181309));
#14352=CARTESIAN_POINT('Ctrl Pts',(3.58910270149602,49.4376309512673,1.2668404425874));
#14353=CARTESIAN_POINT('Ctrl Pts',(1.47372061005109,46.6794679460814,1.10805572336172));
#14354=CARTESIAN_POINT('Ctrl Pts',(-1.98290181661967,46.9604846321805,0.949634426773433));
#14355=CARTESIAN_POINT('Ctrl Pts',(-3.0779493499385,48.9896806575687,0.844141369927042));
#14356=CARTESIAN_POINT('Ctrl Pts',(-3.07857599143262,50.0001497381948,0.791576552822544));
#14357=CARTESIAN_POINT('Origin',(0.,50.,12.2084234471775));
#14358=CARTESIAN_POINT('',(-3.06935579216157,49.998376067411,2.79157655282254));
#14359=CARTESIAN_POINT('',(-3.07814148031383,50.0010564595264,2.70842344717745));
#14360=CARTESIAN_POINT('',(-3.0735,50.0000000000001,12.2084234471775));
#14361=CARTESIAN_POINT('Ctrl Pts',(-3.07814148031383,50.0010564595264,2.70842344717745));
#14362=CARTESIAN_POINT('Ctrl Pts',(-3.07840095523816,50.0592826774211,2.70539570706384));
#14363=CARTESIAN_POINT('Ctrl Pts',(-3.05051243711967,51.1351139926954,2.64943972720834));
#14364=CARTESIAN_POINT('Ctrl Pts',(-1.79264823311626,53.1597984449186,2.54055550761094));
#14365=CARTESIAN_POINT('Ctrl Pts',(1.68282148580427,53.2196308819302,2.38177078838525));
#14366=CARTESIAN_POINT('Ctrl Pts',(3.61769661596932,50.3319453337173,2.22298606915957));
#14367=CARTESIAN_POINT('Ctrl Pts',(2.24062890528198,47.1403675327308,2.06420134993389));
#14368=CARTESIAN_POINT('Ctrl Pts',(-1.1876948837818,46.5667395440464,1.9054166307082));
#14369=CARTESIAN_POINT('Ctrl Pts',(-2.93614411454864,48.4858084944497,1.78682399645606));
#14370=CARTESIAN_POINT('Ctrl Pts',(-3.07554742036879,49.7512558901519,1.72115960194581));
#14371=CARTESIAN_POINT('Ctrl Pts',(-3.07330104137895,49.9971878127024,1.70842344717745));
#14372=CARTESIAN_POINT('Ctrl Pts',(-3.06935579216157,49.998376067411,2.79157655282254));
#14373=CARTESIAN_POINT('Ctrl Pts',(-3.06639561916484,50.6161884641465,2.75968534042121));
#14374=CARTESIAN_POINT('Ctrl Pts',(-2.58560749438489,52.2635918629999,2.67486588827799));
#14375=CARTESIAN_POINT('Ctrl Pts',(0.101753748544503,53.6314673752793,2.53711819639287));
#14376=CARTESIAN_POINT('Ctrl Pts',(3.10637882983628,51.8836985739372,2.37833347716719));
#14377=CARTESIAN_POINT('Ctrl Pts',(3.26716539423699,48.4114345548525,2.2195487579415));
#14378=CARTESIAN_POINT('Ctrl Pts',(0.436916036883408,46.3934765333616,2.06076403871582));
#14379=CARTESIAN_POINT('Ctrl Pts',(-2.46523651005939,47.546842799228,1.9181066370095));
#14380=CARTESIAN_POINT('Ctrl Pts',(-3.06570868289955,49.2908785023193,1.82837747504507));
#14381=CARTESIAN_POINT('Ctrl Pts',(-3.0714204791275,50.0025993512516,1.79157655282254));
#14382=CARTESIAN_POINT('Origin',(0.,50.,12.2084234471775));
#14383=CARTESIAN_POINT('',(-3.07734549507316,49.9982621438963,3.79157655282254));
#14384=CARTESIAN_POINT('',(-3.07017362606608,50.0021532365281,3.70842344717745));
#14385=CARTESIAN_POINT('',(-3.0735,50.0000000000001,12.2084234471775));
#14386=CARTESIAN_POINT('Ctrl Pts',(-3.07017362606608,50.0021532365281,3.70842344717745));
#14387=CARTESIAN_POINT('Ctrl Pts',(-3.07252461422455,50.3659511320327,3.68963181218188));
#14388=CARTESIAN_POINT('Ctrl Pts',(-2.84443426502969,51.7515648716753,3.61791193744441));
#14389=CARTESIAN_POINT('Ctrl Pts',(-0.788934856752224,53.54619447354,3.49326382296504));
#14390=CARTESIAN_POINT('Ctrl Pts',(2.551748227883,52.5858256675908,3.33447910373936));
#14391=CARTESIAN_POINT('Ctrl Pts',(3.5563479740914,49.2581761937472,3.17569438451367));
#14392=CARTESIAN_POINT('Ctrl Pts',(1.30516987545015,46.6096541304332,3.01690966528799));
#14393=CARTESIAN_POINT('Ctrl Pts',(-2.07515983968236,47.0562563206458,2.86115268617591));
#14394=CARTESIAN_POINT('Ctrl Pts',(-3.07386504710643,49.0414241082048,2.75832394680574));
#14395=CARTESIAN_POINT('Ctrl Pts',(-3.07814148031383,50.0010564595264,2.70842344717745));
#14396=CARTESIAN_POINT('Ctrl Pts',(-3.07734549507316,49.9982621438963,3.79157655282254));
#14397=CARTESIAN_POINT('Ctrl Pts',(-3.0711410240522,50.9153404750885,3.74392144553925));
#14398=CARTESIAN_POINT('Ctrl Pts',(-2.14944206797417,52.8617971516187,3.64333809851406));
#14399=CARTESIAN_POINT('Ctrl Pts',(1.160548502562,53.4425334553022,3.48982651174698));
#14400=CARTESIAN_POINT('Ctrl Pts',(3.52177447035456,50.8916355787576,3.33104179252129));
#14401=CARTESIAN_POINT('Ctrl Pts',(2.65887408716728,47.524460054095,3.17225707329561));
#14402=CARTESIAN_POINT('Ctrl Pts',(-0.638181599955106,46.4236004656121,
3.01347235406992));
#14403=CARTESIAN_POINT('Ctrl Pts',(-2.80613642398289,48.1603828111261,2.88657884724557));
#14404=CARTESIAN_POINT('Ctrl Pts',(-3.07130846926525,49.5908363314516,2.81261358016311));
#14405=CARTESIAN_POINT('Ctrl Pts',(-3.06935579216157,49.998376067411,2.79157655282254));
#14406=CARTESIAN_POINT('Origin',(0.,50.,12.2084234471775));
#14407=CARTESIAN_POINT('',(-3.07461570809594,50.002710506979,4.79157655282254));
#14408=CARTESIAN_POINT('',(-3.07035160721926,49.9977623829844,4.70842344717745));
#14409=CARTESIAN_POINT('',(-3.0735,50.0000000000001,12.2084234471775));
#14410=CARTESIAN_POINT('Ctrl Pts',(-3.07035160721926,49.9977623829844,4.70842344717746));
#14411=CARTESIAN_POINT('Ctrl Pts',(-3.06584225025972,50.6666449550227,4.67386791729991));
#14412=CARTESIAN_POINT('Ctrl Pts',(-2.52195697727917,52.3667212082676,4.58638414768047));
#14413=CARTESIAN_POINT('Ctrl Pts',(0.283925502051857,53.621781295074,4.44597213831914));
#14414=CARTESIAN_POINT('Ctrl Pts',(3.19702456896977,51.7253832457192,4.28718741909346));
#14415=CARTESIAN_POINT('Ctrl Pts',(3.18330045542969,48.2494253370868,4.12840269986777));
#14416=CARTESIAN_POINT('Ctrl Pts',(0.255317360099809,46.3760896137859,3.96961798064209));
#14417=CARTESIAN_POINT('Ctrl Pts',(-2.53222545405911,47.6494566272368,3.82962489641198));
#14418=CARTESIAN_POINT('Ctrl Pts',(-3.06590285593096,49.3412833883586,3.74256005192377));
#14419=CARTESIAN_POINT('Ctrl Pts',(-3.07017362606608,50.0021532365281,3.70842344717745));
#14420=CARTESIAN_POINT('Ctrl Pts',(-3.07461570809594,50.002710506979,4.79157655282255));
#14421=CARTESIAN_POINT('Ctrl Pts',(-3.07647553176869,50.205062018161,4.78108579039918));
#14422=CARTESIAN_POINT('Ctrl Pts',(-2.96604334544996,51.4263020184257,4.71766678823391));
#14423=CARTESIAN_POINT('Ctrl Pts',(-1.33190075959052,53.3799334001034,4.60131954632676));
#14424=CARTESIAN_POINT('Ctrl Pts',(2.1176259614783,52.951875625715,4.44253482710107));
#14425=CARTESIAN_POINT('Ctrl Pts',(3.62850109627196,49.8214244786094,4.28375010787539));
#14426=CARTESIAN_POINT('Ctrl Pts',(1.81754341731002,46.8544562713326,4.12496538864971));
#14427=CARTESIAN_POINT('Ctrl Pts',(-1.65734523585442,46.76718138599,3.96618066942402));
#14428=CARTESIAN_POINT('Ctrl Pts',(-3.02743399158457,48.7774471850316,3.85505105748164));
#14429=CARTESIAN_POINT('Ctrl Pts',(-3.07803203213905,49.8967856014863,3.79684968528114));
#14430=CARTESIAN_POINT('Ctrl Pts',(-3.07734549507316,49.9982621438963,3.79157655282254));
#14431=CARTESIAN_POINT('Origin',(0.,50.,12.2084234471775));
#14432=CARTESIAN_POINT('',(-3.06849806069028,50.0000666768364,5.79157655282255));
#14433=CARTESIAN_POINT('',(-3.0782507036788,49.9990828923494,5.70842344717746));
#14434=CARTESIAN_POINT('',(-3.0735,50.0000000000001,12.2084234471775));
#14435=CARTESIAN_POINT('Ctrl Pts',(-3.0782507036788,49.9990828923494,5.70842344717746));
#14436=CARTESIAN_POINT('Ctrl Pts',(-3.07444452114988,50.9666800272788,5.65810402241794));
#14437=CARTESIAN_POINT('Ctrl Pts',(-2.06095094116992,52.9589090168758,5.55485635791654));
#14438=CARTESIAN_POINT('Ctrl Pts',(1.3319009622986,53.3799339145109,5.39868045367324));
#14439=CARTESIAN_POINT('Ctrl Pts',(3.56209487930137,50.7137180890468,5.23989573444756));
#14440=CARTESIAN_POINT('Ctrl Pts',(2.53124977721441,47.3941051431169,5.08111101522187));
#14441=CARTESIAN_POINT('Ctrl Pts',(-0.816912681732443,46.460145891388,4.92232629599619));
#14442=CARTESIAN_POINT('Ctrl Pts',(-2.85131635541723,48.2648648637016,4.79809710664805));
#14443=CARTESIAN_POINT('Ctrl Pts',(-3.07274917158553,49.6421265275098,4.72679615704181));
#14444=CARTESIAN_POINT('Ctrl Pts',(-3.07035160721926,49.9977623829844,4.70842344717746));
#14445=CARTESIAN_POINT('Ctrl Pts',(-3.06849806069028,50.0000666768364,5.79157655282255));
#14446=CARTESIAN_POINT('Ctrl Pts',(-3.0685965252858,50.5090402624651,5.76532189551721));
#14447=CARTESIAN_POINT('Ctrl Pts',(-2.70766479984231,52.0439509300286,5.68613899846998));
#14448=CARTESIAN_POINT('Ctrl Pts',(-0.283925458840122,53.6217807438589,
5.55402786168086));
#14449=CARTESIAN_POINT('Ctrl Pts',(2.889102232167,52.2024980623317,5.39524314245518));
#14450=CARTESIAN_POINT('Ctrl Pts',(3.41720455519345,48.7668647882805,5.23645842322949));
#14451=CARTESIAN_POINT('Ctrl Pts',(0.816912557402795,46.4601464301344,5.07767370400381));
#14452=CARTESIAN_POINT('Ctrl Pts',(-2.3100393678769,47.3323997082042,4.92937974720149));
#14453=CARTESIAN_POINT('Ctrl Pts',(-3.06709230591183,49.1841534450989,4.83401403014107));
#14454=CARTESIAN_POINT('Ctrl Pts',(-3.07461570809594,50.002710506979,4.79157655282255));
#14455=CARTESIAN_POINT('Origin',(0.,50.,12.2084234471775));
#14456=CARTESIAN_POINT('',(-3.07437087614155,49.9972554431979,6.79157655282255));
#14457=CARTESIAN_POINT('',(-3.0730581170342,50.0028093778768,6.70842344717746));
#14458=CARTESIAN_POINT('',(-3.0735,50.0000000000001,12.2084234471775));
#14459=CARTESIAN_POINT('Ctrl Pts',(-3.0730581170342,50.0028093778768,6.70842344717746));
#14460=CARTESIAN_POINT('Ctrl Pts',(-3.07535959640269,50.2568814410373,6.69526836727788));
#14461=CARTESIAN_POINT('Ctrl Pts',(-2.93032368413276,51.5305969754684,6.6291850476364));
#14462=CARTESIAN_POINT('Ctrl Pts',(-1.16054867919063,53.4425339792431,6.51017348825302));
#14463=CARTESIAN_POINT('Ctrl Pts',(2.26314079233676,52.8418492563365,6.35138876902735));
#14464=CARTESIAN_POINT('Ctrl Pts',(3.6149622537802,49.6394984830586,6.19260404980166));
#14465=CARTESIAN_POINT('Ctrl Pts',(1.65734548809325,46.7671808939717,6.03381933057597));
#14466=CARTESIAN_POINT('Ctrl Pts',(-1.81754369393026,46.8544557925985,5.87503461135029));
#14467=CARTESIAN_POINT('Ctrl Pts',(-3.05460283140418,48.8811818580631,5.76656931688412));
#14468=CARTESIAN_POINT('Ctrl Pts',(-3.07844803554526,49.9489177341708,5.71103226215984));
#14469=CARTESIAN_POINT('Ctrl Pts',(-3.0782507036788,49.9990828923494,5.70842344717746));
#14470=CARTESIAN_POINT('Ctrl Pts',(-3.07437087614155,49.9972554431979,6.79157655282255));
#14471=CARTESIAN_POINT('Ctrl Pts',(-3.06689206860327,50.8078980828033,6.74955800063525));
#14472=CARTESIAN_POINT('Ctrl Pts',(-2.32221817630179,52.6518097217997,6.65461120870605));
#14473=CARTESIAN_POINT('Ctrl Pts',(0.788934736670248,53.5461939338473,6.50673617703496));
#14474=CARTESIAN_POINT('Ctrl Pts',(3.40736059977763,51.2600806198138,6.34795145780928));
#14475=CARTESIAN_POINT('Ctrl Pts',(2.90640411768017,47.8203843177281,6.1891667385836));
#14476=CARTESIAN_POINT('Ctrl Pts',(-0.255317321240407,46.3760901653225,
6.03038201935791));
#14477=CARTESIAN_POINT('Ctrl Pts',(-2.69916534238486,47.939674261022,5.89785195743756));
#14478=CARTESIAN_POINT('Ctrl Pts',(-3.06839802497186,49.482971795863,5.81825013525911));
#14479=CARTESIAN_POINT('Ctrl Pts',(-3.06849806069028,50.0000666768364,5.79157655282255));
#14480=CARTESIAN_POINT('Origin',(0.,50.,12.2084234471775));
#14481=CARTESIAN_POINT('',(-3.07751802765106,50.0016205064162,7.79157655282255));
#14482=CARTESIAN_POINT('',(-3.06867630081942,49.9992281639212,7.70842344717746));
#14483=CARTESIAN_POINT('',(-3.0735,50.0000000000001,12.2084234471775));
#14484=CARTESIAN_POINT('Ctrl Pts',(-3.06867630081942,49.9992281639212,7.70842344717746));
#14485=CARTESIAN_POINT('Ctrl Pts',(-3.0674168112757,50.559771360493,7.67950447239591));
#14486=CARTESIAN_POINT('Ctrl Pts',(-2.65206070693095,52.1479727200386,7.59765725787247));
#14487=CARTESIAN_POINT('Ctrl Pts',(-0.101753763996771,53.6314679282393,
7.46288180360713));
#14488=CARTESIAN_POINT('Ctrl Pts',(2.99602565802517,52.0546882429035,7.30409708438145));
#14489=CARTESIAN_POINT('Ctrl Pts',(3.3509930854224,48.5968753391809,7.14531236515576));
#14490=CARTESIAN_POINT('Ctrl Pts',(0.638181697078704,46.4235999212631,6.98652764593008));
#14491=CARTESIAN_POINT('Ctrl Pts',(-2.38571824726309,47.4332550695025,6.84089800660398));
#14492=CARTESIAN_POINT('Ctrl Pts',(-3.06609980834313,49.2346461392885,6.74819660701977));
#14493=CARTESIAN_POINT('Ctrl Pts',(-3.0730581170342,50.0028093778768,6.70842344717746));
#14494=CARTESIAN_POINT('Ctrl Pts',(-3.07751802765106,50.0016205064162,7.79157655282255));
#14495=CARTESIAN_POINT('Ctrl Pts',(-3.07811546112488,50.095021443553,7.78672234549518));
#14496=CARTESIAN_POINT('Ctrl Pts',(-3.03188884220289,51.2062275721529,7.72893989842591));
#14497=CARTESIAN_POINT('Ctrl Pts',(-1.68282122891848,53.2196303903089,7.61822921161475));
#14498=CARTESIAN_POINT('Ctrl Pts',(1.79264795986253,53.1597979648733,7.45944449238905));
#14499=CARTESIAN_POINT('Ctrl Pts',(3.62697790104741,50.2072222411372,7.30065977316339));
#14500=CARTESIAN_POINT('Ctrl Pts',(2.14086931327707,47.0649382107817,7.14187505393769));
#14501=CARTESIAN_POINT('Ctrl Pts',(-1.30516967674285,46.6096546462972,6.98309033471202));
#14502=CARTESIAN_POINT('Ctrl Pts',(-2.96062745118739,48.5573088293533,6.86632416767363));
#14503=CARTESIAN_POINT('Ctrl Pts',(-3.07631267206921,49.7867803683524,6.80248624037714));
#14504=CARTESIAN_POINT('Ctrl Pts',(-3.07437087614155,49.9972554431979,6.79157655282255));
#14505=CARTESIAN_POINT('Origin',(0.,50.,12.2084234471775));
#14506=CARTESIAN_POINT('',(-3.06948424112278,50.0017243562825,8.79157655282255));
#14507=CARTESIAN_POINT('',(-3.0758887284968,49.9975848851305,8.70842344717746));
#14508=CARTESIAN_POINT('',(-3.0735,50.0000000000001,12.2084234471775));
#14509=CARTESIAN_POINT('Ctrl Pts',(-3.0758887284968,49.9975848851305,8.70842344717746));
#14510=CARTESIAN_POINT('Ctrl Pts',(-3.06846894672027,50.8585303398374,8.66374057751394));
#14511=CARTESIAN_POINT('Ctrl Pts',(-2.24296276284576,52.7517665575233,8.56612946810853));
#14512=CARTESIAN_POINT('Ctrl Pts',(0.965959558335722,53.5021163068972,8.41559011896124));
#14513=CARTESIAN_POINT('Ctrl Pts',(3.4663211670797,51.087443472416,8.25680539973554));
#14514=CARTESIAN_POINT('Ctrl Pts',(2.79332321135939,47.6772296827595,8.09802068050987));
#14515=CARTESIAN_POINT('Ctrl Pts',(-0.436916103658114,46.3934759827048,
7.93923596128417));
#14516=CARTESIAN_POINT('Ctrl Pts',(-2.75170116252904,48.0439097412714,7.80937021684004));
#14517=CARTESIAN_POINT('Ctrl Pts',(-3.06972196092315,49.533851011727,7.7324327121378));
#14518=CARTESIAN_POINT('Ctrl Pts',(-3.06867630081942,49.9992281639212,7.70842344717746));
#14519=CARTESIAN_POINT('Ctrl Pts',(-3.06948424112278,50.0017243562825,8.79157655282255));
#14520=CARTESIAN_POINT('Ctrl Pts',(-3.07153463083539,50.4011105484092,8.77095845061321));
#14521=CARTESIAN_POINT('Ctrl Pts',(-2.81347939940506,51.823212235849,8.69741210866198));
#14522=CARTESIAN_POINT('Ctrl Pts',(-0.666391154437672,53.5712334545473,
8.57093752696884));
#14523=CARTESIAN_POINT('Ctrl Pts',(2.63923735448624,52.496466169517,8.41215280774317));
#14524=CARTESIAN_POINT('Ctrl Pts',(3.52870838065631,49.1361979230418,8.25336808851748));
#14525=CARTESIAN_POINT('Ctrl Pts',(1.18769469860156,46.5667400770053,8.0945833692918));
#14526=CARTESIAN_POINT('Ctrl Pts',(-2.13582129838156,47.1228315854216,7.94065285739348));
#14527=CARTESIAN_POINT('Ctrl Pts',(-3.0716012972255,49.0766168185547,7.83965058523707));
#14528=CARTESIAN_POINT('Ctrl Pts',(-3.07751802765106,50.0016205064162,7.79157655282255));
#14529=CARTESIAN_POINT('Origin',(0.,50.,12.2084234471775));
#14530=CARTESIAN_POINT('',(-3.0704093202101,49.9964518649217,9.79157655282255));
#14531=CARTESIAN_POINT('',(-3.07627326766851,50.0022126145262,9.70842344717746));
#14532=CARTESIAN_POINT('',(-3.0735,50.0000000000001,12.2084234471775));
#14533=CARTESIAN_POINT('',(-0.79379928253289,47.0307770462543,10.));
#14534=CARTESIAN_POINT('Ctrl Pts',(-0.79379928253289,47.0307770462543,10.));
#14535=CARTESIAN_POINT('Ctrl Pts',(-1.78123794632762,47.2947612990625,9.94707176025811));
#14536=CARTESIAN_POINT('Ctrl Pts',(-2.87965183287623,48.3360650844884,9.87759727786562));
#14537=CARTESIAN_POINT('Ctrl Pts',(-3.07283314005625,49.6763547812676,9.80812279547314));
#14538=CARTESIAN_POINT('Ctrl Pts',(-3.0704093202101,49.9964518649217,9.79157655282255));
#14539=CARTESIAN_POINT('',(0.795527717319754,47.0254679690975,10.));
#14540=CARTESIAN_POINT('Origin',(0.,50.,10.));
#14541=CARTESIAN_POINT('Ctrl Pts',(0.79552895279625,47.0254641741959,10.));
#14542=CARTESIAN_POINT('Ctrl Pts',(-0.166671812615051,46.7696422359245,
9.94821753066412));
#14543=CARTESIAN_POINT('Ctrl Pts',(-2.23052341514648,47.2443566461646,9.85102534638995));
#14544=CARTESIAN_POINT('Ctrl Pts',(-3.06903578357325,49.12775239834,9.75383316211577));
#14545=CARTESIAN_POINT('Ctrl Pts',(-3.07627326766851,50.0022126145262,9.70842344717746));
#14546=CARTESIAN_POINT('Origin',(-5.55111512312578E-16,7.54951656745106E-14,
4.));
#14547=CARTESIAN_POINT('',(-7.44220860705898,25.9540657903346,4.));
#14548=CARTESIAN_POINT('',(7.44220860705898,25.9540657903346,4.));
#14549=CARTESIAN_POINT('Origin',(-5.55111512312578E-16,7.54951656745106E-14,
4.));
#14550=CARTESIAN_POINT('',(-7.44220860705898,25.9540657903346,0.));
#14551=CARTESIAN_POINT('',(-7.44220860705898,25.9540657903346,4.));
#14552=CARTESIAN_POINT('',(7.44220860705898,25.9540657903346,0.));
#14553=CARTESIAN_POINT('Origin',(-5.55111512312578E-16,7.54951656745106E-14,
0.));
#14554=CARTESIAN_POINT('',(7.44220860705898,25.9540657903346,4.));
#14555=CARTESIAN_POINT('Origin',(-6.89093389542498,24.031542398458,4.));
#14556=CARTESIAN_POINT('',(-6.33965915514315,22.109019014796,4.));
#14557=CARTESIAN_POINT('Origin',(-6.89093389542498,24.031542398458,4.));
#14558=CARTESIAN_POINT('',(-6.33965915514315,22.109019014796,0.));
#14559=CARTESIAN_POINT('',(-6.33965915514315,22.109019014796,4.));
#14560=CARTESIAN_POINT('Origin',(-6.89093389542498,24.031542398458,0.));
#14561=CARTESIAN_POINT('Origin',(0.,-1.06581410364015E-13,4.));
#14562=CARTESIAN_POINT('',(6.33965918379098,22.1090190065813,4.));
#14563=CARTESIAN_POINT('Origin',(0.,-1.06581410364015E-13,4.));
#14564=CARTESIAN_POINT('',(6.33965918379098,22.1090190065813,0.));
#14565=CARTESIAN_POINT('',(6.33965918379098,22.1090190065813,4.));
#14566=CARTESIAN_POINT('Origin',(0.,-1.06581410364015E-13,0.));
#14567=CARTESIAN_POINT('Origin',(6.89093389542498,24.031542398458,4.));
#14568=CARTESIAN_POINT('Origin',(6.89093389542498,24.031542398458,4.));
#14569=CARTESIAN_POINT('Origin',(6.89093389542498,24.031542398458,0.));
#14570=CARTESIAN_POINT('Origin',(0.,50.,12.2084234471775));
#14571=CARTESIAN_POINT('Ctrl Pts',(-3.07627326766851,50.0022126145262,9.70842344717746));
#14572=CARTESIAN_POINT('Ctrl Pts',(-3.07747158401468,50.1469977300918,9.70090492237387));
#14573=CARTESIAN_POINT('Ctrl Pts',(-3.00235625554453,51.3098177813352,9.64045815782839));
#14574=CARTESIAN_POINT('Ctrl Pts',(-1.5190875024664,53.3003399032799,9.52708315354102));
#14575=CARTESIAN_POINT('Ctrl Pts',(1.94901703988696,53.0656764961195,9.36829843431533));
#14576=CARTESIAN_POINT('Ctrl Pts',(3.63280460830591,50.0249606151346,9.20951371508965));
#14577=CARTESIAN_POINT('Ctrl Pts',(1.99083173979432,46.9611289474581,9.05072899586396));
#14578=CARTESIAN_POINT('Ctrl Pts',(-1.4737208527869,46.6794673744635,8.89194427663828));
#14579=CARTESIAN_POINT('Ctrl Pts',(-2.99382331557603,48.6614689264833,8.77784242707612));
#14580=CARTESIAN_POINT('Ctrl Pts',(-3.07725790749334,49.8387138469717,8.71666881725584));
#14581=CARTESIAN_POINT('Ctrl Pts',(-3.0758887284968,49.9975848851305,8.70842344717746));
#14582=CARTESIAN_POINT('Ctrl Pts',(-3.0704093202101,49.9964518649217,9.79157655282255));
#14583=CARTESIAN_POINT('Ctrl Pts',(-3.06507980773682,50.7002836297739,9.75519455573125));
#14584=CARTESIAN_POINT('Ctrl Pts',(-2.47718564593827,52.4386050547508,9.66588431889805));
#14585=CARTESIAN_POINT('Ctrl Pts',(0.409110549274297,53.6089507129763,9.52364584232294));
#14586=CARTESIAN_POINT('Ctrl Pts',(3.25417230454442,51.6147744981929,9.36486112309727));
#14587=CARTESIAN_POINT('Ctrl Pts',(3.12133210059845,48.1406572795451,9.20607640387158));
#14588=CARTESIAN_POINT('Ctrl Pts',(0.130337574092825,46.3695668156037,9.0472916846459));
#14589=CARTESIAN_POINT('Ctrl Pts',(-2.57583048728707,47.7201204800813,8.90912506762955));
#14590=CARTESIAN_POINT('Ctrl Pts',(-3.06627112417646,49.3758557547402,8.82388669035511));
#14591=CARTESIAN_POINT('Ctrl Pts',(-3.06948424112278,50.0017243562825,8.79157655282255));
#14592=CARTESIAN_POINT('Ctrl Pts',(1.91346599666507,51.6359872033749,10.));
#14593=CARTESIAN_POINT('Ctrl Pts',(2.45752652807378,50.9996488965529,9.94707176025811));
#14594=CARTESIAN_POINT('Ctrl Pts',(2.85111340926301,49.1521369412685,9.84121528077433));
#14595=CARTESIAN_POINT('Ctrl Pts',(0.83051951135165,47.140667390072,9.68243056154863));
#14596=CARTESIAN_POINT('Ctrl Pts',(-1.95060983334475,47.7536969022194,9.52364584232296));
#14597=CARTESIAN_POINT('Ctrl Pts',(-2.94584357496186,50.4198377036174,9.36486112309726));
#14598=CARTESIAN_POINT('Ctrl Pts',(-1.24428267039504,52.7033042806271,9.20607640387159));
#14599=CARTESIAN_POINT('Ctrl Pts',(1.59643741594775,52.5110917777716,9.0472916846459));
#14600=CARTESIAN_POINT('Ctrl Pts',(2.97562570405406,50.02044520859,8.88850696542022));
#14601=CARTESIAN_POINT('Ctrl Pts',(1.63068778426296,47.5108645274852,8.72972224619453));
#14602=CARTESIAN_POINT('Ctrl Pts',(-1.20712290447081,47.2801558858669,8.57093752696885));
#14603=CARTESIAN_POINT('Ctrl Pts',(-2.93982996683955,49.5393641766748,8.41215280774316));
#14604=CARTESIAN_POINT('Ctrl Pts',(-1.98117254630264,52.2203049740253,8.25336808851749));
#14605=CARTESIAN_POINT('Ctrl Pts',(0.791216264229766,52.8685790800761,8.09458336929179));
#14606=CARTESIAN_POINT('Ctrl Pts',(2.83925932589008,50.8907235860768,7.93579865006612));
#14607=CARTESIAN_POINT('Ctrl Pts',(2.28800754338613,48.0974217427516,7.77701393084044));
#14608=CARTESIAN_POINT('Ctrl Pts',(-0.357877433206215,47.0459006951226,
7.61822921161474));
#14609=CARTESIAN_POINT('Ctrl Pts',(-2.67613148900519,48.6988078365273,7.45944449238906));
#14610=CARTESIAN_POINT('Ctrl Pts',(-2.54443139563822,51.5429353767203,7.30065977316338));
#14611=CARTESIAN_POINT('Ctrl Pts',(-0.0833463806285565,52.9745308310859,
7.14187505393769));
#14612=CARTESIAN_POINT('Ctrl Pts',(2.45404086353615,51.6829925659703,6.98309033471202));
#14613=CARTESIAN_POINT('Ctrl Pts',(2.74479423866956,48.8507023479382,6.82430561548632));
#14614=CARTESIAN_POINT('Ctrl Pts',(0.522733828662967,47.0705751754612,6.66552089626065));
#14615=CARTESIAN_POINT('Ctrl Pts',(-2.1778807656371,47.9722880226893,6.50673617703496));
#14616=CARTESIAN_POINT('Ctrl Pts',(-2.88468149617291,50.730337696803,6.34795145780928));
#14617=CARTESIAN_POINT('Ctrl Pts',(-0.950603969371205,52.8197752701299,
6.18916673858359));
#14618=CARTESIAN_POINT('Ctrl Pts',(1.85373578809429,52.3277551660412,6.03038201935791));
#14619=CARTESIAN_POINT('Ctrl Pts',(2.96101105381215,49.7047136590531,5.87159730013223));
#14620=CARTESIAN_POINT('Ctrl Pts',(1.35752961323402,47.3520019198223,5.71281258090655));
#14621=CARTESIAN_POINT('Ctrl Pts',(-1.48874776296386,47.4234886799631,5.55402786168086));
#14622=CARTESIAN_POINT('Ctrl Pts',(-2.97210115507541,49.8537289918586,5.39524314245518));
#14623=CARTESIAN_POINT('Ctrl Pts',(-1.7345450364046,52.4178779953631,5.23645842322949));
#14624=CARTESIAN_POINT('Ctrl Pts',(1.09095840982161,52.7684996355234,5.07767370400381));
#14625=CARTESIAN_POINT('Ctrl Pts',(2.91770745360052,50.5846055927038,4.91888898477812));
#14626=CARTESIAN_POINT('Ctrl Pts',(2.07334352176257,47.8655147869845,4.76010426555244));
#14627=CARTESIAN_POINT('Ctrl Pts',(-0.669132154306629,47.1005099338114,
4.60131954632676));
#14628=CARTESIAN_POINT('Ctrl Pts',(-2.79902839661656,48.9899403390338,4.44253482710108));
#14629=CARTESIAN_POINT('Ctrl Pts',(-2.3664603795149,51.8040636784796,4.28375010787539));
#14630=CARTESIAN_POINT('Ctrl Pts',(0.232563023073223,52.966596521994,4.12496538864971));
#14631=CARTESIAN_POINT('Ctrl Pts',(2.61867881971088,51.4132592552783,3.96618066942402));
#14632=CARTESIAN_POINT('Ctrl Pts',(2.60743741550163,48.5661064864539,3.80739595019834));
#14633=CARTESIAN_POINT('Ctrl Pts',(0.209130129836104,47.03165954212,3.64861123097265));
#14634=CARTESIAN_POINT('Ctrl Pts',(-2.3806323344251,48.2146792532123,3.48982651174698));
#14635=CARTESIAN_POINT('Ctrl Pts',(-2.79096522383464,51.0321306143504,3.33104179252129));
#14636=CARTESIAN_POINT('Ctrl Pts',(-0.646215552911574,52.9046834511589,
3.17225707329561));
#14637=CARTESIAN_POINT('Ctrl Pts',(2.09013377702796,52.1180465652057,3.01347235406992));
#14638=CARTESIAN_POINT('Ctrl Pts',(2.91300017074186,49.3923730495392,2.85468763484424));
#14639=CARTESIAN_POINT('Ctrl Pts',(1.06906301006856,47.2229719451328,2.69590291561855));
#14640=CARTESIAN_POINT('Ctrl Pts',(-1.75358363974743,47.5958941989475,2.53711819639287));
#14641=CARTESIAN_POINT('Ctrl Pts',(-2.97085350739628,50.1697355043467,2.37833347716719));
#14642=CARTESIAN_POINT('Ctrl Pts',(-1.46835592219625,52.5881869481317,2.21954875794151));
#14643=CARTESIAN_POINT('Ctrl Pts',(1.37839697104677,52.6371956223391,2.06076403871582));
#14644=CARTESIAN_POINT('Ctrl Pts',(2.96325076645608,50.2718960070387,1.90197931949014));
#14645=CARTESIAN_POINT('Ctrl Pts',(1.83529632960708,47.65767862816,1.74319460026445));
#14646=CARTESIAN_POINT('Ctrl Pts',(-0.972839391547319,47.1878206611801,
1.58440988103877));
#14647=CARTESIAN_POINT('Ctrl Pts',(-2.89036104794741,49.2924607089264,1.42562516181309));
#14648=CARTESIAN_POINT('Ctrl Pts',(-2.16179635093426,52.0448525943808,1.2668404425874));
#14649=CARTESIAN_POINT('Ctrl Pts',(0.545840261212082,52.9251933476136,1.10805572336172));
#14650=CARTESIAN_POINT('Ctrl Pts',(2.75380262558533,51.1276121450193,0.949271004136036));
#14651=CARTESIAN_POINT('Ctrl Pts',(2.44063792264946,48.297633157129,0.790486284910355));
#14652=CARTESIAN_POINT('Ctrl Pts',(-0.106759426258933,47.0263159609106,
0.631701565684669));
#14653=CARTESIAN_POINT('Ctrl Pts',(-2.55667952108434,48.4770150283179,0.472916846458987));
#14654=CARTESIAN_POINT('Ctrl Pts',(-2.665488928155,51.3226590034494,0.314132127233303));
#14655=CARTESIAN_POINT('Ctrl Pts',(-0.335102051433244,52.9560891299428,
0.155347408007618));
#14656=CARTESIAN_POINT('Ctrl Pts',(2.30407741786964,51.8859408488594,-0.00343731121806405));
#14657=CARTESIAN_POINT('Ctrl Pts',(2.82987294110782,49.0837366230026,-0.162222030443749));
#14658=CARTESIAN_POINT('Ctrl Pts',(1.45900977058067,47.7841423687619,-0.268078509927538));
#14659=CARTESIAN_POINT('Ctrl Pts',(0.650199997975087,47.5679131979649,-0.321006749669432));
#14660=CARTESIAN_POINT('Ctrl Pts',(2.0543315503421,51.7564253212268,10.1070022498898));
#14661=CARTESIAN_POINT('Ctrl Pts',(2.6384447339141,51.0732410562991,10.0540740101479));
#14662=CARTESIAN_POINT('Ctrl Pts',(3.06100669698896,49.0897189524364,9.94821753066413));
#14663=CARTESIAN_POINT('Ctrl Pts',(0.891660702786476,46.9301690211716,9.78943281143844));
#14664=CARTESIAN_POINT('Ctrl Pts',(-2.09420984226096,47.5883285444086,9.63064809221277));
#14665=CARTESIAN_POINT('Ctrl Pts',(-3.16271070871609,50.4507453187398,9.47186337298707));
#14666=CARTESIAN_POINT('Ctrl Pts',(-1.33588428108549,52.9023161548447,9.3130786537614));
#14667=CARTESIAN_POINT('Ctrl Pts',(1.71396395726082,52.6959533505542,9.1542939345357));
#14668=CARTESIAN_POINT('Ctrl Pts',(3.19468533880467,50.0219503441049,8.99550921531003));
#14669=CARTESIAN_POINT('Ctrl Pts',(1.75073576944008,47.3276193341428,8.83672449608433));
#14670=CARTESIAN_POINT('Ctrl Pts',(-1.29598888724284,47.0799263820657,8.67793977685867));
#14671=CARTESIAN_POINT('Ctrl Pts',(-3.15625439074724,49.5054530852787,8.51915505763297));
#14672=CARTESIAN_POINT('Ctrl Pts',(-2.12702252124395,52.3837594017721,8.3603703384073));
#14673=CARTESIAN_POINT('Ctrl Pts',(0.849464028931752,53.0797581556832,8.2015856191816));
#14674=CARTESIAN_POINT('Ctrl Pts',(3.04827993961995,50.9562968815233,8.04280089995593));
#14675=CARTESIAN_POINT('Ctrl Pts',(2.45644609937722,47.9573577227543,7.88401618073025));
#14676=CARTESIAN_POINT('Ctrl Pts',(-0.384223656690181,46.8284257909833,
7.72523146150455));
#14677=CARTESIAN_POINT('Ctrl Pts',(-2.87314295645131,48.603016662361,7.56644674227888));
#14678=CARTESIAN_POINT('Ctrl Pts',(-2.73174736465177,51.65652320452,7.40766202305319));
#14679=CARTESIAN_POINT('Ctrl Pts',(-0.0894821750846268,53.1935098634703,
7.2488773038275));
#14680=CARTESIAN_POINT('Ctrl Pts',(2.63470246169916,51.806891124948,7.09009258460183));
#14681=CARTESIAN_POINT('Ctrl Pts',(2.94686052092051,48.7660933450191,6.93130786537613));
#14682=CARTESIAN_POINT('Ctrl Pts',(0.561216451468212,46.8549167573952,6.77252314615046));
#14683=CARTESIAN_POINT('Ctrl Pts',(-2.33821200770187,47.8230119075771,6.61373842692477));
#14684=CARTESIAN_POINT('Ctrl Pts',(-3.09704599956545,50.7841037026847,6.45495370769909));
#14685=CARTESIAN_POINT('Ctrl Pts',(-1.02058553931101,53.027361506501,6.2961689884734));
#14686=CARTESIAN_POINT('Ctrl Pts',(1.99020412284178,52.4991198628063,6.13738426924772));
#14687=CARTESIAN_POINT('Ctrl Pts',(3.17899478713483,49.6829752670549,5.97859955002203));
#14688=CARTESIAN_POINT('Ctrl Pts',(1.45746823818709,47.1570615778722,5.81981483079636));
#14689=CARTESIAN_POINT('Ctrl Pts',(-1.59834640661933,47.2338110508415,5.66103011157067));
#14690=CARTESIAN_POINT('Ctrl Pts',(-3.19090131955365,49.842960811716,5.50224539234499));
#14691=CARTESIAN_POINT('Ctrl Pts',(-1.86223878552621,52.5958773552336,5.3434606731193));
#14692=CARTESIAN_POINT('Ctrl Pts',(1.17127259398061,52.9723110618525,5.18467595389362));
#14693=CARTESIAN_POINT('Ctrl Pts',(3.13250326216747,50.6276430914849,5.02589123466794));
#14694=CARTESIAN_POINT('Ctrl Pts',(2.22597894024652,47.7083782390286,4.86710651544225));
#14695=CARTESIAN_POINT('Ctrl Pts',(-0.718392330115233,46.8870552530037,
4.70832179621657));
#14696=CARTESIAN_POINT('Ctrl Pts',(-3.00508728950221,48.9155817595572,4.54953707699089));
#14697=CARTESIAN_POINT('Ctrl Pts',(-2.54067447696744,51.9368752514998,4.3907523577652));
#14698=CARTESIAN_POINT('Ctrl Pts',(0.249683849399434,53.184991446354,4.23196763853952));
#14699=CARTESIAN_POINT('Ctrl Pts',(2.81146073613051,51.5173005854253,4.07318291931383));
#14700=CARTESIAN_POINT('Ctrl Pts',(2.79939176214431,48.4605461033315,3.91439820008815));
#14701=CARTESIAN_POINT('Ctrl Pts',(0.224525873257339,46.8131362326752,3.75561348086247));
#14702=CARTESIAN_POINT('Ctrl Pts',(-2.55588974295742,48.083247497474,3.59682876163679));
#14703=CARTESIAN_POINT('Ctrl Pts',(-2.9964305220077,51.108114013434,3.4380440424111));
#14704=CARTESIAN_POINT('Ctrl Pts',(-0.693788654191789,53.1185204586193,
3.27925932318542));
#14705=CARTESIAN_POINT('Ctrl Pts',(2.2440052606463,52.2739729326674,3.12047460395973));
#14706=CARTESIAN_POINT('Ctrl Pts',(3.12744943852504,49.3476407642752,2.96168988473405));
#14707=CARTESIAN_POINT('Ctrl Pts',(1.14776529852909,47.0185326735663,2.80290516550837));
#14708=CARTESIAN_POINT('Ctrl Pts',(-1.88267897290858,47.418908720578,2.64412044628268));
#14709=CARTESIAN_POINT('Ctrl Pts',(-3.18956182253859,50.1822310939418,2.485335727057));
#14710=CARTESIAN_POINT('Ctrl Pts',(-1.57645335916959,52.7787241137273,2.32655100783132));
#14711=CARTESIAN_POINT('Ctrl Pts',(1.47987180929927,52.8313407088695,2.16776628860563));
#14712=CARTESIAN_POINT('Ctrl Pts',(3.1813993829605,50.2919124492648,2.00898156937995));
#14713=CARTESIAN_POINT('Ctrl Pts',(1.97040718816538,47.4852415963503,1.85019685015426));
#14714=CARTESIAN_POINT('Ctrl Pts',(-1.04445788895881,46.9807936221355,1.69141213092858));
#14715=CARTESIAN_POINT('Ctrl Pts',(-3.10314366862385,49.2403730762436,1.5326274117029));
#14716=CARTESIAN_POINT('Ctrl Pts',(-2.32094349044031,52.1953905675652,1.37384269247722));
#14717=CARTESIAN_POINT('Ctrl Pts',(0.586023933536996,53.1405402527805,1.21505797325153));
#14718=CARTESIAN_POINT('Ctrl Pts',(2.95653208732984,51.2106247041231,1.05627325402585));
#14719=CARTESIAN_POINT('Ctrl Pts',(2.62031282301266,48.1723083024932,0.897488534800166));
#14720=CARTESIAN_POINT('Ctrl Pts',(-0.114618842478724,46.8073992676655,
0.73870381557448));
#14721=CARTESIAN_POINT('Ctrl Pts',(-2.74489717268617,48.3648959095816,0.579919096348797));
#14722=CARTESIAN_POINT('Ctrl Pts',(-2.86171691147896,51.4200305235974,0.421134377123114));
#14723=CARTESIAN_POINT('Ctrl Pts',(-0.359771596695991,53.1737105210381,
0.262349657897429));
#14724=CARTESIAN_POINT('Ctrl Pts',(2.47369900599749,52.0247800560049,0.103564938671747));
#14725=CARTESIAN_POINT('Ctrl Pts',(3.03820254789444,49.0162831390423,-0.0552197805539385));
#14726=CARTESIAN_POINT('Ctrl Pts',(1.56641916249631,47.6210153455288,-0.161076260037727));
#14727=CARTESIAN_POINT('Ctrl Pts',(0.698066426161006,47.3888678140614,-0.214004499779622));
#14728=CARTESIAN_POINT('Ctrl Pts',(2.19519710401913,51.8768634390787,10.2140044997796));
#14729=CARTESIAN_POINT('Ctrl Pts',(2.81936293975442,51.1468332160454,10.1610762600377));
#14730=CARTESIAN_POINT('Ctrl Pts',(3.27089998471491,49.0273009636042,10.0552197805539));
#14731=CARTESIAN_POINT('Ctrl Pts',(0.952801894221302,46.7196706522712,9.89643506132826));
#14732=CARTESIAN_POINT('Ctrl Pts',(-2.23780985117717,47.4229601865978,9.73765034210257));
#14733=CARTESIAN_POINT('Ctrl Pts',(-3.37957784247032,50.4816529338621,9.57886562287689));
#14734=CARTESIAN_POINT('Ctrl Pts',(-1.42748589177595,53.1013280290623,9.42008090365121));
#14735=CARTESIAN_POINT('Ctrl Pts',(1.83149049857389,52.8808149233369,9.26129618442552));
#14736=CARTESIAN_POINT('Ctrl Pts',(3.41374497355529,50.0234554796197,9.10251146519984));
#14737=CARTESIAN_POINT('Ctrl Pts',(1.8707837546172,47.1443741408005,8.94372674597414));
#14738=CARTESIAN_POINT('Ctrl Pts',(-1.38485487001487,46.8796968782645,8.78494202674848));
#14739=CARTESIAN_POINT('Ctrl Pts',(-3.37267881465492,49.4715419938827,8.62615730752278));
#14740=CARTESIAN_POINT('Ctrl Pts',(-2.27287249618527,52.5472138295189,8.46737258829712));
#14741=CARTESIAN_POINT('Ctrl Pts',(0.907711793633738,53.2909372312903,8.30858786907141));
#14742=CARTESIAN_POINT('Ctrl Pts',(3.25730055334983,51.0218701769695,8.14980314984575));
#14743=CARTESIAN_POINT('Ctrl Pts',(2.6248846553683,47.817293702757,7.99101843062005));
#14744=CARTESIAN_POINT('Ctrl Pts',(-0.410569880174145,46.610950886844,7.83223371139438));
#14745=CARTESIAN_POINT('Ctrl Pts',(-3.07015442389744,48.5072254881948,7.67344899216868));
#14746=CARTESIAN_POINT('Ctrl Pts',(-2.91906333366532,51.7701110323196,7.51466427294301));
#14747=CARTESIAN_POINT('Ctrl Pts',(-0.0956179695407002,53.4124888958548,
7.35587955371731));
#14748=CARTESIAN_POINT('Ctrl Pts',(2.81536405986217,51.9307896839258,7.19709483449164));
#14749=CARTESIAN_POINT('Ctrl Pts',(3.14892680317145,48.6814843421,7.03831011526595));
#14750=CARTESIAN_POINT('Ctrl Pts',(0.599699074273457,46.6392583393292,6.87952539604027));
#14751=CARTESIAN_POINT('Ctrl Pts',(-2.49854324976665,47.6737357924649,6.72074067681458));
#14752=CARTESIAN_POINT('Ctrl Pts',(-3.30941050295798,50.8378697085665,6.5619559575889));
#14753=CARTESIAN_POINT('Ctrl Pts',(-1.09056710925082,53.2349477428722,6.40317123836322));
#14754=CARTESIAN_POINT('Ctrl Pts',(2.12667245758927,52.6704845595713,6.24438651913753));
#14755=CARTESIAN_POINT('Ctrl Pts',(3.39697852045751,49.6612368750568,6.08560179991185));
#14756=CARTESIAN_POINT('Ctrl Pts',(1.55740686314017,46.9621212359219,5.92681708068617));
#14757=CARTESIAN_POINT('Ctrl Pts',(-1.7079450502748,47.04413342172,5.76803236146048));
#14758=CARTESIAN_POINT('Ctrl Pts',(-3.40970148403189,49.8321926315735,5.6092476422348));
#14759=CARTESIAN_POINT('Ctrl Pts',(-1.98993253464782,52.7738767151041,5.45046292300911));
#14760=CARTESIAN_POINT('Ctrl Pts',(1.2515867781396,53.1761224881817,5.29167820378343));
#14761=CARTESIAN_POINT('Ctrl Pts',(3.34729907073442,50.6706805902658,5.13289348455775));
#14762=CARTESIAN_POINT('Ctrl Pts',(2.37861435873046,47.5512416910727,4.97410876533206));
#14763=CARTESIAN_POINT('Ctrl Pts',(-0.767652505923838,46.6736005721958,
4.81532404610638));
#14764=CARTESIAN_POINT('Ctrl Pts',(-3.21114618238785,48.8412231800806,4.6565393268807));
#14765=CARTESIAN_POINT('Ctrl Pts',(-2.71488857441997,52.0696868245199,4.49775460765501));
#14766=CARTESIAN_POINT('Ctrl Pts',(0.266804675725645,53.403386370714,4.33896988842933));
#14767=CARTESIAN_POINT('Ctrl Pts',(3.00424265255014,51.6213419155723,4.18018516920365));
#14768=CARTESIAN_POINT('Ctrl Pts',(2.991346108787,48.3549857202091,4.02140044997796));
#14769=CARTESIAN_POINT('Ctrl Pts',(0.239921616678574,46.5946129232305,3.86261573075228));
#14770=CARTESIAN_POINT('Ctrl Pts',(-2.73114715148974,47.9518157417356,3.7038310115266));
#14771=CARTESIAN_POINT('Ctrl Pts',(-3.20189582018077,51.1840974125176,3.54504629230091));
#14772=CARTESIAN_POINT('Ctrl Pts',(-0.741361755472007,53.3323574660797,
3.38626157307523));
#14773=CARTESIAN_POINT('Ctrl Pts',(2.39787674426465,52.4298993001291,3.22747685384955));
#14774=CARTESIAN_POINT('Ctrl Pts',(3.34189870630822,49.3029084790112,3.06869213462386));
#14775=CARTESIAN_POINT('Ctrl Pts',(1.22646758698962,46.8140934019998,2.90990741539818));
#14776=CARTESIAN_POINT('Ctrl Pts',(-2.01177430606972,47.2419232422086,2.75112269617249));
#14777=CARTESIAN_POINT('Ctrl Pts',(-3.40827013768091,50.1947266835369,2.59233797694681));
#14778=CARTESIAN_POINT('Ctrl Pts',(-1.68455079614292,52.9692612793229,2.43355325772113));
#14779=CARTESIAN_POINT('Ctrl Pts',(1.58134664755177,53.0254857953999,2.27476853849544));
#14780=CARTESIAN_POINT('Ctrl Pts',(3.39954799946491,50.311928891491,2.11598381926976));
#14781=CARTESIAN_POINT('Ctrl Pts',(2.10551804672368,47.3128045645405,1.95719910004408));
#14782=CARTESIAN_POINT('Ctrl Pts',(-1.11607638637031,46.773766583091,1.79841438081839));
#14783=CARTESIAN_POINT('Ctrl Pts',(-3.31592628930028,49.1882854435608,1.63962966159271));
#14784=CARTESIAN_POINT('Ctrl Pts',(-2.48009062994636,52.3459285407497,1.48084494236703));
#14785=CARTESIAN_POINT('Ctrl Pts',(0.626207605861911,53.3558871579475,1.32206022314134));
#14786=CARTESIAN_POINT('Ctrl Pts',(3.15926154907436,51.2936372632267,1.16327550391566));
#14787=CARTESIAN_POINT('Ctrl Pts',(2.79998772337587,48.0469834478575,1.00449078468998));
#14788=CARTESIAN_POINT('Ctrl Pts',(-0.122478258698513,46.5884825744204,
0.845706065464291));
#14789=CARTESIAN_POINT('Ctrl Pts',(-2.93311482428801,48.2527767908454,0.686921346238607));
#14790=CARTESIAN_POINT('Ctrl Pts',(-3.05794489480291,51.5174020437455,0.528136627012925));
#14791=CARTESIAN_POINT('Ctrl Pts',(-0.384441141958736,53.3913319121335,
0.369351907787239));
#14792=CARTESIAN_POINT('Ctrl Pts',(2.64332059412533,52.1636192631504,0.210567188561558));
#14793=CARTESIAN_POINT('Ctrl Pts',(3.24653215468106,48.9488296550819,0.0517824693358721));
#14794=CARTESIAN_POINT('Ctrl Pts',(1.67382855441195,47.4578883222956,-0.0540740101479162));
#14795=CARTESIAN_POINT('Ctrl Pts',(0.745932854346925,47.2098224301578,-0.107002249889811));
#14796=CARTESIAN_POINT('Ctrl Pts',(2.33606265769616,51.9973015569306,10.3210067496694));
#14797=CARTESIAN_POINT('Ctrl Pts',(3.00028114559474,51.2204253757916,10.2680785099275));
#14798=CARTESIAN_POINT('Ctrl Pts',(3.48079327244086,48.9648829747721,10.1622220304438));
#14799=CARTESIAN_POINT('Ctrl Pts',(1.01394308565613,46.5091722833709,10.0034373112181));
#14800=CARTESIAN_POINT('Ctrl Pts',(-2.38140986009338,47.257591828787,9.84465259199239));
#14801=CARTESIAN_POINT('Ctrl Pts',(-3.59644497622454,50.5125605489844,9.6858678727667));
#14802=CARTESIAN_POINT('Ctrl Pts',(-1.5190875024664,53.3003399032799,9.52708315354102));
#14803=CARTESIAN_POINT('Ctrl Pts',(1.94901703988696,53.0656764961195,9.36829843431533));
#14804=CARTESIAN_POINT('Ctrl Pts',(3.63280460830591,50.0249606151346,9.20951371508965));
#14805=CARTESIAN_POINT('Ctrl Pts',(1.99083173979432,46.9611289474581,9.05072899586396));
#14806=CARTESIAN_POINT('Ctrl Pts',(-1.4737208527869,46.6794673744635,8.89194427663828));
#14807=CARTESIAN_POINT('Ctrl Pts',(-3.58910323856261,49.4376309024865,8.7331595574126));
#14808=CARTESIAN_POINT('Ctrl Pts',(-2.41872247112658,52.7106682572659,8.57437483818691));
#14809=CARTESIAN_POINT('Ctrl Pts',(0.965959558335722,53.5021163068972,8.41559011896124));
#14810=CARTESIAN_POINT('Ctrl Pts',(3.4663211670797,51.087443472416,8.25680539973554));
#14811=CARTESIAN_POINT('Ctrl Pts',(2.79332321135939,47.6772296827595,8.09802068050987));
#14812=CARTESIAN_POINT('Ctrl Pts',(-0.436916103658114,46.3934759827048,
7.93923596128417));
#14813=CARTESIAN_POINT('Ctrl Pts',(-3.26716589134357,48.4114343140284,7.7804512420585));
#14814=CARTESIAN_POINT('Ctrl Pts',(-3.10637930267888,51.8836988601192,7.62166652283282));
#14815=CARTESIAN_POINT('Ctrl Pts',(-0.101753763996771,53.6314679282393,
7.46288180360713));
#14816=CARTESIAN_POINT('Ctrl Pts',(2.99602565802517,52.0546882429035,7.30409708438145));
#14817=CARTESIAN_POINT('Ctrl Pts',(3.3509930854224,48.5968753391809,7.14531236515576));
#14818=CARTESIAN_POINT('Ctrl Pts',(0.638181697078704,46.4235999212631,6.98652764593008));
#14819=CARTESIAN_POINT('Ctrl Pts',(-2.65887449183142,47.5244596773528,6.8277429267044));
#14820=CARTESIAN_POINT('Ctrl Pts',(-3.52177500635052,50.8916357144483,6.66895820747871));
#14821=CARTESIAN_POINT('Ctrl Pts',(-1.16054867919063,53.4425339792431,6.51017348825302));
#14822=CARTESIAN_POINT('Ctrl Pts',(2.26314079233676,52.8418492563365,6.35138876902735));
#14823=CARTESIAN_POINT('Ctrl Pts',(3.6149622537802,49.6394984830586,6.19260404980166));
#14824=CARTESIAN_POINT('Ctrl Pts',(1.65734548809325,46.7671808939717,6.03381933057597));
#14825=CARTESIAN_POINT('Ctrl Pts',(-1.81754369393026,46.8544557925985,5.87503461135029));
#14826=CARTESIAN_POINT('Ctrl Pts',(-3.62850164851013,49.8214244514309,5.71624989212461));
#14827=CARTESIAN_POINT('Ctrl Pts',(-2.11762628376943,52.9518760749746,5.55746517289892));
#14828=CARTESIAN_POINT('Ctrl Pts',(1.3319009622986,53.3799339145109,5.39868045367324));
#14829=CARTESIAN_POINT('Ctrl Pts',(3.56209487930137,50.7137180890468,5.23989573444756));
#14830=CARTESIAN_POINT('Ctrl Pts',(2.53124977721441,47.3941051431169,5.08111101522187));
#14831=CARTESIAN_POINT('Ctrl Pts',(-0.816912681732443,46.460145891388,4.92232629599619));
#14832=CARTESIAN_POINT('Ctrl Pts',(-3.41720507527349,48.766864600604,4.76354157677051));
#14833=CARTESIAN_POINT('Ctrl Pts',(-2.88910267187251,52.2024983975401,4.60475685754483));
#14834=CARTESIAN_POINT('Ctrl Pts',(0.283925502051857,53.621781295074,4.44597213831914));
#14835=CARTESIAN_POINT('Ctrl Pts',(3.19702456896977,51.7253832457192,4.28718741909346));
#14836=CARTESIAN_POINT('Ctrl Pts',(3.18330045542969,48.2494253370868,4.12840269986777));
#14837=CARTESIAN_POINT('Ctrl Pts',(0.255317360099809,46.3760896137859,3.96961798064209));
#14838=CARTESIAN_POINT('Ctrl Pts',(-2.90640456002206,47.8203839859972,3.81083326141641));
#14839=CARTESIAN_POINT('Ctrl Pts',(-3.40736111835383,51.2600808116012,3.65204854219072));
#14840=CARTESIAN_POINT('Ctrl Pts',(-0.788934856752224,53.54619447354,3.49326382296504));
#14841=CARTESIAN_POINT('Ctrl Pts',(2.551748227883,52.5858256675908,3.33447910373936));
#14842=CARTESIAN_POINT('Ctrl Pts',(3.5563479740914,49.2581761937472,3.17569438451367));
#14843=CARTESIAN_POINT('Ctrl Pts',(1.30516987545015,46.6096541304332,3.01690966528799));
#14844=CARTESIAN_POINT('Ctrl Pts',(-2.14086963923087,47.0649377638391,2.8581249460623));
#14845=CARTESIAN_POINT('Ctrl Pts',(-3.62697845282322,50.2072222731319,2.69934022683662));
#14846=CARTESIAN_POINT('Ctrl Pts',(-1.79264823311626,53.1597984449186,2.54055550761094));
#14847=CARTESIAN_POINT('Ctrl Pts',(1.68282148580427,53.2196308819302,2.38177078838525));
#14848=CARTESIAN_POINT('Ctrl Pts',(3.61769661596932,50.3319453337173,2.22298606915957));
#14849=CARTESIAN_POINT('Ctrl Pts',(2.24062890528198,47.1403675327308,2.06420134993389));
#14850=CARTESIAN_POINT('Ctrl Pts',(-1.1876948837818,46.5667395440464,1.9054166307082));
#14851=CARTESIAN_POINT('Ctrl Pts',(-3.52870890997671,49.136197810878,1.74663191148252));
#14852=CARTESIAN_POINT('Ctrl Pts',(-2.63923776945242,52.4964665139341,1.58784719225684));
#14853=CARTESIAN_POINT('Ctrl Pts',(0.666391278186825,53.5712340631145,1.42906247303115));
#14854=CARTESIAN_POINT('Ctrl Pts',(3.36199101081887,51.3766498223304,1.27027775380547));
#14855=CARTESIAN_POINT('Ctrl Pts',(2.97966262373907,47.9216585932218,1.11149303457979));
#14856=CARTESIAN_POINT('Ctrl Pts',(-0.130337674918302,46.3695658811752,
0.952708315354101));
#14857=CARTESIAN_POINT('Ctrl Pts',(-3.12133247588985,48.1406576721092,0.793923596128419));
#14858=CARTESIAN_POINT('Ctrl Pts',(-3.25417287812687,51.6147735638935,0.635138876902735));
#14859=CARTESIAN_POINT('Ctrl Pts',(-0.409110687221481,53.6089533032289,
0.47635415767705));
#14860=CARTESIAN_POINT('Ctrl Pts',(2.81294218225317,52.3024584702958,0.317569438451368));
#14861=CARTESIAN_POINT('Ctrl Pts',(3.45486176146768,48.8813761711215,0.158784719225683));
#14862=CARTESIAN_POINT('Ctrl Pts',(1.78123794632758,47.2947612990625,0.0529282397418946));
#14863=CARTESIAN_POINT('Ctrl Pts',(0.793799282532844,47.0307770462543,0.));
#14864=CARTESIAN_POINT('Ctrl Pts',(0.793799282532844,47.0307770462543,0.));
#14865=CARTESIAN_POINT('Ctrl Pts',(0.886857327319536,47.0648180947248,2.20021361319926E-16));
#14866=CARTESIAN_POINT('Ctrl Pts',(0.97784812376529,47.1036280421655,1.56093797443782E-15));
#14867=CARTESIAN_POINT('Ctrl Pts',(1.06656383114865,47.146878310404,8.32667268468867E-16));
#14868=CARTESIAN_POINT('Ctrl Pts',(1.15724741706422,47.191087949614,8.82421707898277E-17));
#14869=CARTESIAN_POINT('Ctrl Pts',(1.24555453014161,47.2399377005581,4.94586033878426E-16));
#14870=CARTESIAN_POINT('Ctrl Pts',(1.33123425142126,47.2931221802054,2.77555756156289E-16));
#14871=CARTESIAN_POINT('Ctrl Pts',(1.414183141195,47.3446115346763,6.74427875860411E-17));
#14872=CARTESIAN_POINT('Ctrl Pts',(1.49466977869018,47.4001645661104,-2.35200004845136E-15));
#14873=CARTESIAN_POINT('Ctrl Pts',(1.57243277080527,47.4595348565004,-3.10862446895044E-15));
#14874=CARTESIAN_POINT('Ctrl Pts',(1.64047538890598,47.5114838605917,-3.77067083688713E-15));
#14875=CARTESIAN_POINT('Ctrl Pts',(1.70643241927354,47.5663561703348,-2.05196266536534E-15));
#14876=CARTESIAN_POINT('Ctrl Pts',(1.77010348490124,47.6239996814536,-3.66373598126302E-15));
#14877=CARTESIAN_POINT('Ctrl Pts',(1.78344332214389,47.6360766751216,-4.00142145101522E-15));
#14878=CARTESIAN_POINT('Ctrl Pts',(1.79668458295983,47.648277209747,-1.16810055785692E-16));
#14879=CARTESIAN_POINT('Ctrl Pts',(1.80980825419109,47.6605835920549,-1.11022302462516E-16));
#14880=CARTESIAN_POINT('Ctrl Pts',(1.88223649041001,47.7285012919949,-7.90802675333328E-17));
#14881=CARTESIAN_POINT('Ctrl Pts',(1.95119902453439,47.7997400265197,-4.2204114024801E-15));
#14882=CARTESIAN_POINT('Ctrl Pts',(2.01645648006057,47.87400881514,-3.58046925441613E-15));
#14883=CARTESIAN_POINT('Ctrl Pts',(2.08135180887242,47.9478654713505,-2.94407827373316E-15));
#14884=CARTESIAN_POINT('Ctrl Pts',(2.14258355052389,48.0247194439553,-4.09959586981255E-15));
#14885=CARTESIAN_POINT('Ctrl Pts',(2.19987267902198,48.1043113151144,-3.33066907387547E-15));
#14886=CARTESIAN_POINT('Ctrl Pts',(2.25572844020942,48.1819118069438,-2.58098073665603E-15));
#14887=CARTESIAN_POINT('Ctrl Pts',(2.30783667769722,48.2621156470778,4.07626245988852E-17));
#14888=CARTESIAN_POINT('Ctrl Pts',(2.35589192627243,48.3446965327013,-4.71844785465692E-16));
#14889=CARTESIAN_POINT('Ctrl Pts',(2.37661944628707,48.3803158877216,-6.92946135823573E-16));
#14890=CARTESIAN_POINT('Ctrl Pts',(2.39659231188801,48.4163775922232,-5.2526661233185E-16));
#14891=CARTESIAN_POINT('Ctrl Pts',(2.41578302796428,48.4528638195851,-3.60822483003176E-16));
#14892=CARTESIAN_POINT('Ctrl Pts',(2.42944452020578,48.4788376451601,-2.43757950963101E-16));
#14893=CARTESIAN_POINT('Ctrl Pts',(2.44270960171289,48.5050266109815,-2.2454156296485E-15));
#14894=CARTESIAN_POINT('Ctrl Pts',(2.45556775734007,48.5314242897153,-2.44249065417534E-15));
#14895=CARTESIAN_POINT('Ctrl Pts',(2.46118164896502,48.5429495591131,-2.52853392987966E-15));
#14896=CARTESIAN_POINT('Ctrl Pts',(2.46671705248137,48.5545128335615,1.92714193980372E-16));
#14897=CARTESIAN_POINT('Ctrl Pts',(2.47216939081917,48.566105287244,1.94289029309402E-16));
#14898=CARTESIAN_POINT('Ctrl Pts',(2.51239835158546,48.6516378304363,2.05908628963686E-16));
#14899=CARTESIAN_POINT('Ctrl Pts',(2.54817131413657,48.7388840438779,-2.2713001230117E-15));
#14900=CARTESIAN_POINT('Ctrl Pts',(2.57923728625574,48.8276067891984,-1.83186799063151E-15));
#14901=CARTESIAN_POINT('Ctrl Pts',(2.60961659647764,48.9143684650762,-1.4021487782457E-15));
#14902=CARTESIAN_POINT('Ctrl Pts',(2.63549491455905,49.0025427959324,5.44463455921423E-16));
#14903=CARTESIAN_POINT('Ctrl Pts',(2.65658840962129,49.0919168481172,1.47104550762833E-15));
#14904=CARTESIAN_POINT('Ctrl Pts',(2.66032086411668,49.107731419475,1.63500246848459E-15));
#14905=CARTESIAN_POINT('Ctrl Pts',(2.66390337128728,49.1235835631294,1.68482728082412E-15));
#14906=CARTESIAN_POINT('Ctrl Pts',(2.66733418587856,49.1394721050097,1.9151347174784E-15));
#14907=CARTESIAN_POINT('Ctrl Pts',(2.68744489614248,49.2326073805454,3.26407681196226E-15));
#14908=CARTESIAN_POINT('Ctrl Pts',(2.70234744457541,49.3269943616445,-3.40775973016887E-15));
#14909=CARTESIAN_POINT('Ctrl Pts',(2.71212035484507,49.4222239812899,-3.05311331771918E-15));
#14910=CARTESIAN_POINT('Ctrl Pts',(2.71539798866634,49.4541620441108,-2.93417217900389E-15));
#14911=CARTESIAN_POINT('Ctrl Pts',(2.7180982270661,49.4861947652343,9.25563036540978E-16));
#14912=CARTESIAN_POINT('Ctrl Pts',(2.72022280748871,49.5183062439642,7.7715611723761E-16));
#14913=CARTESIAN_POINT('Ctrl Pts',(2.7214113229284,49.5362697853089,6.94135529703041E-16));
#14914=CARTESIAN_POINT('Ctrl Pts',(2.72241968039311,49.5542579679131,3.13605320939017E-15));
#14915=CARTESIAN_POINT('Ctrl Pts',(2.72324810469235,49.5722679631563,3.27515792264421E-15));
#14916=CARTESIAN_POINT('Ctrl Pts',(2.72382227638594,49.584750491107,3.37156985656304E-15));
#14917=CARTESIAN_POINT('Ctrl Pts',(2.72430989801868,49.597241968614,5.36242468914633E-16));
#14918=CARTESIAN_POINT('Ctrl Pts',(2.72471091953202,49.6097319728608,4.9960036108132E-16));
#14919=CARTESIAN_POINT('Ctrl Pts',(2.72770312507896,49.7029256264329,2.26196778816368E-16));
#14920=CARTESIAN_POINT('Ctrl Pts',(2.72588562145581,49.7961843599269,5.65648183417809E-16));
#14921=CARTESIAN_POINT('Ctrl Pts',(2.71939754410297,49.8891328761941,1.23512311489549E-15));
#14922=CARTESIAN_POINT('Ctrl Pts',(2.71289651492916,49.9822669408875,1.90593448534879E-15));
#14923=CARTESIAN_POINT('Ctrl Pts',(2.70170586262138,50.075090530546,4.03808733020254E-15));
#14924=CARTESIAN_POINT('Ctrl Pts',(2.68591451135734,50.1672140980482,5.39845945723982E-15));
#14925=CARTESIAN_POINT('Ctrl Pts',(2.67034644847316,50.2580350460475,6.7395960367198E-15));
#14926=CARTESIAN_POINT('Ctrl Pts',(2.65030640580631,50.348176475764,4.44579026743949E-15));
#14927=CARTESIAN_POINT('Ctrl Pts',(2.6258365433358,50.4372399806273,4.7045700668491E-15));
#14928=CARTESIAN_POINT('Ctrl Pts',(2.61632310862035,50.4718662414028,4.80517891703474E-15));
#14929=CARTESIAN_POINT('Ctrl Pts',(2.60613967316216,50.5063292337113,2.00838248105005E-15));
#14930=CARTESIAN_POINT('Ctrl Pts',(2.59528714815,50.5406040828628,1.99840144432528E-15));
#14931=CARTESIAN_POINT('Ctrl Pts',(2.5894827385199,50.5589357857857,1.99306314511668E-15));
#14932=CARTESIAN_POINT('Ctrl Pts',(2.58348691601437,50.5772136532266,4.83308587950495E-15));
#14933=CARTESIAN_POINT('Ctrl Pts',(2.5772997243422,50.5954337650825,4.94049245958195E-15));
#14934=CARTESIAN_POINT('Ctrl Pts',(2.5718499055314,50.6114824530153,5.03509861234435E-15));
#14935=CARTESIAN_POINT('Ctrl Pts',(2.5662511329767,50.6274874088124,-7.84775819580116E-16));
#14936=CARTESIAN_POINT('Ctrl Pts',(2.56050956139753,50.6434295339054,-4.85722573273506E-16));
#14937=CARTESIAN_POINT('Ctrl Pts',(2.5280829941685,50.7334655778652,1.20323489468014E-15));
#14938=CARTESIAN_POINT('Ctrl Pts',(2.49106539149493,50.821622868814,6.21849611564327E-15));
#14939=CARTESIAN_POINT('Ctrl Pts',(2.4495298227146,50.9074566537128,7.32747196252603E-15));
#14940=CARTESIAN_POINT('Ctrl Pts',(2.41837814612936,50.971831992387,8.15920384768811E-15));
#14941=CARTESIAN_POINT('Ctrl Pts',(2.3846839652608,51.0348998219571,5.7554240688827E-15));
#14942=CARTESIAN_POINT('Ctrl Pts',(2.34846073836671,51.0964553528622,5.51642065360625E-15));
#14943=CARTESIAN_POINT('Ctrl Pts',(2.33352951737538,51.1218285543683,5.41790340052968E-15));
#14944=CARTESIAN_POINT('Ctrl Pts',(2.31816842560509,51.1469446029168,3.64806198334203E-15));
#14945=CARTESIAN_POINT('Ctrl Pts',(2.30237774790741,51.1717882500971,3.51801920928096E-15));
#14946=CARTESIAN_POINT('Ctrl Pts',(2.29294436447259,51.1866298961782,3.44033138776168E-15));
#14947=CARTESIAN_POINT('Ctrl Pts',(2.28336234355129,51.2013669072614,6.3072103585326E-15));
#14948=CARTESIAN_POINT('Ctrl Pts',(2.27363372765336,51.2159939545931,6.13398221105399E-15));
#14949=CARTESIAN_POINT('Ctrl Pts',(2.22610568566997,51.2874527239563,5.28769587880953E-15));
#14950=CARTESIAN_POINT('Ctrl Pts',(2.17506913351012,51.3563092996365,3.87680889073946E-15));
#14951=CARTESIAN_POINT('Ctrl Pts',(2.12055847790166,51.4222108593004,3.96210841913103E-15));
#14952=CARTESIAN_POINT('Ctrl Pts',(2.06897016170881,51.4845794083408,4.04283500355103E-15));
#14953=CARTESIAN_POINT('Ctrl Pts',(2.01426976271456,51.5443015075236,-7.75360004353403E-16));
#14954=CARTESIAN_POINT('Ctrl Pts',(1.95646265307235,51.601042205567,1.35308431126191E-16));
#14955=CARTESIAN_POINT('Ctrl Pts',(1.94349660304568,51.613769061034,3.33958961373067E-16));
#14956=CARTESIAN_POINT('Ctrl Pts',(1.93037416921141,51.6263457638983,-1.91541932274788E-17));
#14957=CARTESIAN_POINT('Ctrl Pts',(1.91709858156531,51.6387709851531,5.55111512312578E-17));
#14958=CARTESIAN_POINT('Ctrl Pts',(1.91346599666507,51.6359872033749,10.));
#14959=CARTESIAN_POINT('Ctrl Pts',(1.97508237614856,51.5780829367082,10.));
#14960=CARTESIAN_POINT('Ctrl Pts',(2.03332776396516,51.5170283993854,10.));
#14961=CARTESIAN_POINT('Ctrl Pts',(2.08820515281575,51.4532083325515,10.));
#14962=CARTESIAN_POINT('Ctrl Pts',(2.14453492336427,51.3876992076378,10.));
#14963=CARTESIAN_POINT('Ctrl Pts',(2.19731649744598,51.3192757995672,10.));
#14964=CARTESIAN_POINT('Ctrl Pts',(2.24652756554328,51.2483056584003,10.));
#14965=CARTESIAN_POINT('Ctrl Pts',(2.29742972651859,51.1748966939174,10.));
#14966=CARTESIAN_POINT('Ctrl Pts',(2.3445123533709,51.0987624345107,10.));
#14967=CARTESIAN_POINT('Ctrl Pts',(2.38771583441218,51.0202656546028,10.));
#14968=CARTESIAN_POINT('Ctrl Pts',(2.40661735736774,50.985923313393,10.));
#14969=CARTESIAN_POINT('Ctrl Pts',(2.42477589363752,50.9511282648287,10.));
#14970=CARTESIAN_POINT('Ctrl Pts',(2.44218400642212,50.915908799321,10.));
#14971=CARTESIAN_POINT('Ctrl Pts',(2.45169083165477,50.8966749336221,10.));
#14972=CARTESIAN_POINT('Ctrl Pts',(2.46097382245344,50.8773144696349,10.));
#14973=CARTESIAN_POINT('Ctrl Pts',(2.47003156402945,50.8578318865754,10.));
#14974=CARTESIAN_POINT('Ctrl Pts',(2.47868023930483,50.8392291771701,10.));
#14975=CARTESIAN_POINT('Ctrl Pts',(2.48712604040155,50.8205091346798,10.));
#14976=CARTESIAN_POINT('Ctrl Pts',(2.49535364052389,50.8017084231113,10.));
#14977=CARTESIAN_POINT('Ctrl Pts',(2.53191898243085,50.7181537490415,10.));
#14978=CARTESIAN_POINT('Ctrl Pts',(2.56422392604051,50.6329156432926,10.));
#14979=CARTESIAN_POINT('Ctrl Pts',(2.59224406717849,50.546392863989,10.));
#14980=CARTESIAN_POINT('Ctrl Pts',(2.62072600083341,50.4584441256999,10.));
#14981=CARTESIAN_POINT('Ctrl Pts',(2.64478122692469,50.3691672645249,10.));
#14982=CARTESIAN_POINT('Ctrl Pts',(2.6643450084389,50.2789439546436,10.));
#14983=CARTESIAN_POINT('Ctrl Pts',(2.68356990503497,50.1902834979848,10.));
#14984=CARTESIAN_POINT('Ctrl Pts',(2.69845787026654,50.1007081883537,10.));
#14985=CARTESIAN_POINT('Ctrl Pts',(2.70890477495091,50.0105573646828,10.));
#14986=CARTESIAN_POINT('Ctrl Pts',(2.71303564023117,49.9749103554738,10.));
#14987=CARTESIAN_POINT('Ctrl Pts',(2.7164716351295,49.9391731818997,10.));
#14988=CARTESIAN_POINT('Ctrl Pts',(2.7192042931916,49.9033662888073,10.));
#14989=CARTESIAN_POINT('Ctrl Pts',(2.72082178426693,49.8821717856182,10.));
#14990=CARTESIAN_POINT('Ctrl Pts',(2.72219283242366,49.8609528514772,10.));
#14991=CARTESIAN_POINT('Ctrl Pts',(2.72331547946922,49.8397137034055,10.));
#14992=CARTESIAN_POINT('Ctrl Pts',(2.72406272622749,49.825576682685,10.));
#14993=CARTESIAN_POINT('Ctrl Pts',(2.72469984227435,49.8114307112021,10.));
#14994=CARTESIAN_POINT('Ctrl Pts',(2.72522589886129,49.7972915862557,10.));
#14995=CARTESIAN_POINT('Ctrl Pts',(2.72876702640459,49.7021146679759,10.));
#14996=CARTESIAN_POINT('Ctrl Pts',(2.72728895308013,49.6070864076313,10.));
#14997=CARTESIAN_POINT('Ctrl Pts',(2.72073289392688,49.5126053984232,10.));
#14998=CARTESIAN_POINT('Ctrl Pts',(2.71419948325485,49.4184507821463,10.));
#14999=CARTESIAN_POINT('Ctrl Pts',(2.70262347017024,49.3248386892842,10.));
#15000=CARTESIAN_POINT('Ctrl Pts',(2.68589868103377,49.2321456940246,10.));
#15001=CARTESIAN_POINT('Ctrl Pts',(2.68396182243872,49.221411135693,10.));
#15002=CARTESIAN_POINT('Ctrl Pts',(2.68195585483714,49.2106888933147,10.));
#15003=CARTESIAN_POINT('Ctrl Pts',(2.67988056808785,49.199979545295,10.));
#15004=CARTESIAN_POINT('Ctrl Pts',(2.66233627408987,49.1094436469436,10.));
#15005=CARTESIAN_POINT('Ctrl Pts',(2.63984221727701,49.0198289846102,10.));
#15006=CARTESIAN_POINT('Ctrl Pts',(2.61267377634981,48.9313735730564,10.));
#15007=CARTESIAN_POINT('Ctrl Pts',(2.60192598368317,48.8963807508268,10.));
#15008=CARTESIAN_POINT('Ctrl Pts',(2.5904460787386,48.8615693998425,10.));
#15009=CARTESIAN_POINT('Ctrl Pts',(2.57824891659478,48.8269545976856,10.));
#15010=CARTESIAN_POINT('Ctrl Pts',(2.57231002899096,48.8101003969286,10.));
#15011=CARTESIAN_POINT('Ctrl Pts',(2.56620107697497,48.7932927979567,10.));
#15012=CARTESIAN_POINT('Ctrl Pts',(2.55992367518301,48.7765335691397,10.));
#15013=CARTESIAN_POINT('Ctrl Pts',(2.55466427682359,48.7624921769418,10.));
#15014=CARTESIAN_POINT('Ctrl Pts',(2.5492894967777,48.7484924666187,10.));
#15015=CARTESIAN_POINT('Ctrl Pts',(2.54380264072253,48.734540236572,10.));
#15016=CARTESIAN_POINT('Ctrl Pts',(2.50957844436993,48.6475133753102,10.));
#15017=CARTESIAN_POINT('Ctrl Pts',(2.47097567284871,48.562274017746,10.));
#15018=CARTESIAN_POINT('Ctrl Pts',(2.42832689037754,48.4790541200089,10.));
#15019=CARTESIAN_POINT('Ctrl Pts',(2.38409691699032,48.3927488693328,10.));
#15020=CARTESIAN_POINT('Ctrl Pts',(2.33551523257715,48.308614870025,10.));
#15021=CARTESIAN_POINT('Ctrl Pts',(2.2828968139237,48.2269143645578,10.));
#15022=CARTESIAN_POINT('Ctrl Pts',(2.22970003533411,48.1443158408617,10.));
#15023=CARTESIAN_POINT('Ctrl Pts',(2.17237687628308,48.0642037829466,10.));
#15024=CARTESIAN_POINT('Ctrl Pts',(2.11120119278049,47.9868645265092,10.));
#15025=CARTESIAN_POINT('Ctrl Pts',(2.08739174172464,47.9567642458843,10.));
#15026=CARTESIAN_POINT('Ctrl Pts',(2.06299821502567,47.9270842051726,10.));
#15027=CARTESIAN_POINT('Ctrl Pts',(2.03803489359285,47.8978423233543,10.));
#15028=CARTESIAN_POINT('Ctrl Pts',(2.01823053305732,47.8746436167309,10.));
#15029=CARTESIAN_POINT('Ctrl Pts',(1.9980675313089,47.8517206920118,10.));
#15030=CARTESIAN_POINT('Ctrl Pts',(1.97755259625766,47.8290828275254,10.));
#15031=CARTESIAN_POINT('Ctrl Pts',(1.9658214299723,47.8161376950172,10.));
#15032=CARTESIAN_POINT('Ctrl Pts',(1.95397995403824,47.8032911219115,10.));
#15033=CARTESIAN_POINT('Ctrl Pts',(1.94203528977052,47.7905504717426,10.));
#15034=CARTESIAN_POINT('Ctrl Pts',(1.87297907510553,47.716892388659,10.));
#15035=CARTESIAN_POINT('Ctrl Pts',(1.80042221874533,47.6467115453198,10.));
#15036=CARTESIAN_POINT('Ctrl Pts',(1.72467678835325,47.5802968989121,10.));
#15037=CARTESIAN_POINT('Ctrl Pts',(1.66041809926708,47.5239539869742,10.));
#15038=CARTESIAN_POINT('Ctrl Pts',(1.59386353521053,47.4703215800399,10.));
#15039=CARTESIAN_POINT('Ctrl Pts',(1.52517876205432,47.4195910301052,10.));
#15040=CARTESIAN_POINT('Ctrl Pts',(1.50256045600412,47.4028851570014,10.));
#15041=CARTESIAN_POINT('Ctrl Pts',(1.47971097867339,47.3864941045494,10.));
#15042=CARTESIAN_POINT('Ctrl Pts',(1.45663577987822,47.370425142175,10.));
#15043=CARTESIAN_POINT('Ctrl Pts',(1.43994825627114,47.3588043890302,10.));
#15044=CARTESIAN_POINT('Ctrl Pts',(1.4231416418667,47.3473515143883,10.));
#15045=CARTESIAN_POINT('Ctrl Pts',(1.40623277255848,47.3360788992253,10.));
#15046=CARTESIAN_POINT('Ctrl Pts',(1.31987534930084,47.2785071017792,10.));
#15047=CARTESIAN_POINT('Ctrl Pts',(1.23076881304987,47.2255738593114,10.));
#15048=CARTESIAN_POINT('Ctrl Pts',(1.1392218397819,47.1776007658582,10.));
#15049=CARTESIAN_POINT('Ctrl Pts',(1.04767486651393,47.129627672405,10.));
#15050=CARTESIAN_POINT('Ctrl Pts',(0.95368681063774,47.0866138170145,10.));
#15051=CARTESIAN_POINT('Ctrl Pts',(0.857528305927518,47.0489215422574,10.));
#15052=CARTESIAN_POINT('Ctrl Pts',(0.836959977015811,47.0408591549837,10.));
#15053=CARTESIAN_POINT('Ctrl Pts',(0.816292224819087,47.0330404248373,10.));
#15054=CARTESIAN_POINT('Ctrl Pts',(0.795528952796256,47.0254641741959,10.));
#15055=CARTESIAN_POINT('Ctrl Pts',(-2.51945660451951,49.9980217824357,8.38741669750802));
#15056=CARTESIAN_POINT('Ctrl Pts',(-2.52057809732048,49.8678907140886,8.3956620675864));
#15057=CARTESIAN_POINT('Ctrl Pts',(-2.51136663771178,49.7379189147974,8.40390743766478));
#15058=CARTESIAN_POINT('Ctrl Pts',(-2.49126921968861,49.6096529277652,8.41215280774316));
#15059=CARTESIAN_POINT('Ctrl Pts',(-2.36226094604997,48.7862947464054,8.46508104748506));
#15060=CARTESIAN_POINT('Ctrl Pts',(-1.78469192526039,48.0332253161362,8.51800928722695));
#15061=CARTESIAN_POINT('Ctrl Pts',(-1.0229389667433,47.6951420412712,8.57093752696885));
#15062=CARTESIAN_POINT('Ctrl Pts',(-0.261186008226218,47.3570587664063,
8.62386576671074));
#15063=CARTESIAN_POINT('Ctrl Pts',(0.684750888018369,47.4339616469457,8.67679400645263));
#15064=CARTESIAN_POINT('Ctrl Pts',(1.38187565610585,47.8906765340663,8.72972224619453));
#15065=CARTESIAN_POINT('Ctrl Pts',(2.07900042419332,48.3473914211868,8.78265048593643));
#15066=CARTESIAN_POINT('Ctrl Pts',(2.52731306412369,49.1839183148884,8.83557872567832));
#15067=CARTESIAN_POINT('Ctrl Pts',(2.52160466940449,50.0172895232695,8.88850696542022));
#15068=CARTESIAN_POINT('Ctrl Pts',(2.51589627468529,50.8506607316505,8.94143520516211));
#15069=CARTESIAN_POINT('Ctrl Pts',(2.05616684531652,51.680876254711,8.994363444904));
#15070=CARTESIAN_POINT('Ctrl Pts',(1.35284878290834,52.1280194333839,9.0472916846459));
#15071=CARTESIAN_POINT('Ctrl Pts',(0.649530720500157,52.5751626120567,9.10021992438779));
#15072=CARTESIAN_POINT('Ctrl Pts',(-0.297375974947443,52.6392334463419,
9.15314816412969));
#15073=CARTESIAN_POINT('Ctrl Pts',(-1.05442280676571,52.2906911006495,9.20607640387158));
#15074=CARTESIAN_POINT('Ctrl Pts',(-1.81146963858398,51.9421487549572,9.25900464361348));
#15075=CARTESIAN_POINT('Ctrl Pts',(-2.37865660677292,51.1809932292873,9.31193288335537));
#15076=CARTESIAN_POINT('Ctrl Pts',(-2.49637780059787,50.3560586662194,9.36486112309726));
#15077=CARTESIAN_POINT('Ctrl Pts',(-2.51310024819857,50.2388756462662,9.37237964790085));
#15078=CARTESIAN_POINT('Ctrl Pts',(-2.52075311949145,50.1204056565824,9.37989817270443));
#15079=CARTESIAN_POINT('Ctrl Pts',(-2.51977158007336,50.0018123497868,9.38741669750802));
#15080=CARTESIAN_POINT('Ctrl Pts',(-0.79379928253289,47.0307770462543,10.));
#15081=CARTESIAN_POINT('Ctrl Pts',(-1.78123794632762,47.2947612990625,9.94707176025811));
#15082=CARTESIAN_POINT('Ctrl Pts',(-3.45486289525881,48.881369057802,9.84121528077431));
#15083=CARTESIAN_POINT('Ctrl Pts',(-2.81294119083295,52.3024617009106,9.68243056154864));
#15084=CARTESIAN_POINT('Ctrl Pts',(0.409110549274297,53.6089507129763,9.52364584232294));
#15085=CARTESIAN_POINT('Ctrl Pts',(3.25417230454442,51.6147744981929,9.36486112309727));
#15086=CARTESIAN_POINT('Ctrl Pts',(3.12133210059845,48.1406572795451,9.20607640387158));
#15087=CARTESIAN_POINT('Ctrl Pts',(0.130337574092825,46.3695668156037,9.0472916846459));
#15088=CARTESIAN_POINT('Ctrl Pts',(-2.97966211384112,47.921658696003,8.88850696542022));
#15089=CARTESIAN_POINT('Ctrl Pts',(-3.36199053548259,51.3766497311158,8.72972224619453));
#15090=CARTESIAN_POINT('Ctrl Pts',(-0.666391154437672,53.5712334545473,
8.57093752696884));
#15091=CARTESIAN_POINT('Ctrl Pts',(2.63923735448624,52.496466169517,8.41215280774317));
#15092=CARTESIAN_POINT('Ctrl Pts',(3.52870838065631,49.1361979230418,8.25336808851748));
#15093=CARTESIAN_POINT('Ctrl Pts',(1.18769469860156,46.5667400770053,8.0945833692918));
#15094=CARTESIAN_POINT('Ctrl Pts',(-2.24062856177748,47.1403679623332,7.93579865006611));
#15095=CARTESIAN_POINT('Ctrl Pts',(-3.61769606676686,50.3319452862105,7.77701393084044));
#15096=CARTESIAN_POINT('Ctrl Pts',(-1.68282122891848,53.2196303903089,7.61822921161475));
#15097=CARTESIAN_POINT('Ctrl Pts',(1.79264795986253,53.1597979648733,7.45944449238905));
#15098=CARTESIAN_POINT('Ctrl Pts',(3.62697790104741,50.2072222411372,7.30065977316339));
#15099=CARTESIAN_POINT('Ctrl Pts',(2.14086931327707,47.0649382107817,7.14187505393769));
#15100=CARTESIAN_POINT('Ctrl Pts',(-1.30516967674285,46.6096546462972,6.98309033471202));
#15101=CARTESIAN_POINT('Ctrl Pts',(-3.556347432871,49.2581763067165,6.82430561548633));
#15102=CARTESIAN_POINT('Ctrl Pts',(-2.55174783950134,52.5858252740066,6.66552089626065));
#15103=CARTESIAN_POINT('Ctrl Pts',(0.788934736670248,53.5461939338473,6.50673617703496));
#15104=CARTESIAN_POINT('Ctrl Pts',(3.40736059977763,51.2600806198138,6.34795145780928));
#15105=CARTESIAN_POINT('Ctrl Pts',(2.90640411768017,47.8203843177281,6.1891667385836));
#15106=CARTESIAN_POINT('Ctrl Pts',(-0.255317321240407,46.3760901653225,
6.03038201935791));
#15107=CARTESIAN_POINT('Ctrl Pts',(-3.18329997094959,48.2494256035161,5.87159730013223));
#15108=CARTESIAN_POINT('Ctrl Pts',(-3.19702408239961,51.7253829831247,5.71281258090654));
#15109=CARTESIAN_POINT('Ctrl Pts',(-0.283925458840122,53.6217807438589,
5.55402786168086));
#15110=CARTESIAN_POINT('Ctrl Pts',(2.889102232167,52.2024980623317,5.39524314245518));
#15111=CARTESIAN_POINT('Ctrl Pts',(3.41720455519345,48.7668647882805,5.23645842322949));
#15112=CARTESIAN_POINT('Ctrl Pts',(0.816912557402795,46.4601464301344,5.07767370400381));
#15113=CARTESIAN_POINT('Ctrl Pts',(-2.53124939197203,47.3941055397199,4.91888898477813));
#15114=CARTESIAN_POINT('Ctrl Pts',(-3.56209433716996,50.7137179804228,4.76010426555244));
#15115=CARTESIAN_POINT('Ctrl Pts',(-1.33190075959052,53.3799334001034,4.60131954632676));
#15116=CARTESIAN_POINT('Ctrl Pts',(2.1176259614783,52.951875625715,4.44253482710107));
#15117=CARTESIAN_POINT('Ctrl Pts',(3.62850109627196,49.8214244786094,4.28375010787539));
#15118=CARTESIAN_POINT('Ctrl Pts',(1.81754341731002,46.8544562713326,4.12496538864971));
#15119=CARTESIAN_POINT('Ctrl Pts',(-1.65734523585442,46.76718138599,3.96618066942402));
#15120=CARTESIAN_POINT('Ctrl Pts',(-3.61496170360255,49.6394985379234,3.80739595019834));
#15121=CARTESIAN_POINT('Ctrl Pts',(-2.26314044789927,52.8418488238258,3.64861123097266));
#15122=CARTESIAN_POINT('Ctrl Pts',(1.160548502562,53.4425334553022,3.48982651174698));
#15123=CARTESIAN_POINT('Ctrl Pts',(3.52177447035456,50.8916355787576,3.33104179252129));
#15124=CARTESIAN_POINT('Ctrl Pts',(2.65887408716728,47.524460054095,3.17225707329561));
#15125=CARTESIAN_POINT('Ctrl Pts',(-0.638181599955106,46.4236004656121,
3.01347235406992));
#15126=CARTESIAN_POINT('Ctrl Pts',(-3.35099257541117,48.5968755526526,2.85468763484424));
#15127=CARTESIAN_POINT('Ctrl Pts',(-2.9960252020633,52.054687930335,2.69590291561856));
#15128=CARTESIAN_POINT('Ctrl Pts',(0.101753748544503,53.6314673752793,2.53711819639287));
#15129=CARTESIAN_POINT('Ctrl Pts',(3.10637882983628,51.8836985739372,2.37833347716719));
#15130=CARTESIAN_POINT('Ctrl Pts',(3.26716539423699,48.4114345548525,2.2195487579415));
#15131=CARTESIAN_POINT('Ctrl Pts',(0.436916036883408,46.3934765333616,2.06076403871582));
#15132=CARTESIAN_POINT('Ctrl Pts',(-2.79332278567043,47.6772300330011,1.90197931949014));
#15133=CARTESIAN_POINT('Ctrl Pts',(-3.46632064065236,51.0874433129551,1.74319460026445));
#15134=CARTESIAN_POINT('Ctrl Pts',(-0.965959409052926,53.5021157627911,
1.58440988103877));
#15135=CARTESIAN_POINT('Ctrl Pts',(2.41872209844688,52.7106678650022,1.42562516181309));
#15136=CARTESIAN_POINT('Ctrl Pts',(3.58910270149602,49.4376309512673,1.2668404425874));
#15137=CARTESIAN_POINT('Ctrl Pts',(1.47372061005109,46.6794679460814,1.10805572336172));
#15138=CARTESIAN_POINT('Ctrl Pts',(-1.99083139973657,46.9611292918785,0.949271004136037));
#15139=CARTESIAN_POINT('Ctrl Pts',(-3.63280412987848,50.0249608192598,0.790486284910355));
#15140=CARTESIAN_POINT('Ctrl Pts',(-1.94901659367837,53.0656756689436,0.631701565684669));
#15141=CARTESIAN_POINT('Ctrl Pts',(1.51908697082356,53.300340014212,0.472916846458987));
#15142=CARTESIAN_POINT('Ctrl Pts',(3.59644503276003,50.5125594541255,0.314132127233302));
#15143=CARTESIAN_POINT('Ctrl Pts',(2.38140827918422,47.2575938852802,0.155347408007618));
#15144=CARTESIAN_POINT('Ctrl Pts',(-1.01394043867063,46.5091701825966,-0.00343731121806435));
#15145=CARTESIAN_POINT('Ctrl Pts',(-3.4807982360798,48.9648881946463,-0.162222030443749));
#15146=CARTESIAN_POINT('Ctrl Pts',(-3.00028114559473,51.2204253757917,-0.268078509927538));
#15147=CARTESIAN_POINT('Ctrl Pts',(-2.33606265769613,51.9973015569307,-0.321006749669432));
#15148=CARTESIAN_POINT('Ctrl Pts',(-0.745932854346969,47.2098224301579,
10.1070022498898));
#15149=CARTESIAN_POINT('Ctrl Pts',(-1.67382855441198,47.4578883222957,10.0540740101479));
#15150=CARTESIAN_POINT('Ctrl Pts',(-3.24653322010411,48.9488229706986,9.94821753066412));
#15151=CARTESIAN_POINT('Ctrl Pts',(-2.64331966248816,52.1636222989576,9.78943281143846));
#15152=CARTESIAN_POINT('Ctrl Pts',(0.384441012329826,53.3913294780743,9.63064809221275));
#15153=CARTESIAN_POINT('Ctrl Pts',(3.05794435580772,51.5174029217061,9.47186337298709));
#15154=CARTESIAN_POINT('Ctrl Pts',(2.93311447162684,48.2527764219532,9.31307865376139));
#15155=CARTESIAN_POINT('Ctrl Pts',(0.122478163952854,46.5884834525023,9.15429393453571));
#15156=CARTESIAN_POINT('Ctrl Pts',(-2.79998724422497,48.0469835444409,8.99550921531002));
#15157=CARTESIAN_POINT('Ctrl Pts',(-3.15926110240105,51.2936371775124,8.83672449608434));
#15158=CARTESIAN_POINT('Ctrl Pts',(-0.626207489574883,53.3558865860772,
8.67793977685865));
#15159=CARTESIAN_POINT('Ctrl Pts',(2.48009024000282,52.3459282171011,8.51915505763298));
#15160=CARTESIAN_POINT('Ctrl Pts',(3.31592579189812,49.1882855489611,8.36037033840729));
#15161=CARTESIAN_POINT('Ctrl Pts',(1.11607621235651,46.7737670839123,8.20158561918161));
#15162=CARTESIAN_POINT('Ctrl Pts',(-2.10551772393265,47.3128049682377,8.04280089995592));
#15163=CARTESIAN_POINT('Ctrl Pts',(-3.39954748337958,50.311928846849,7.88401618073025));
#15164=CARTESIAN_POINT('Ctrl Pts',(-1.5813464061563,53.0254853334235,7.72523146150455));
#15165=CARTESIAN_POINT('Ctrl Pts',(1.6845505393665,52.9692608282246,7.56644674227887));
#15166=CARTESIAN_POINT('Ctrl Pts',(3.40826961917741,50.1947266534715,7.40766202305319));
#15167=CARTESIAN_POINT('Ctrl Pts',(2.01177399977108,47.2419236622003,7.24887730382751));
#15168=CARTESIAN_POINT('Ctrl Pts',(-1.22646740026446,46.814093886757,7.09009258460182));
#15169=CARTESIAN_POINT('Ctrl Pts',(-3.34189819772363,49.3029085851684,6.93130786537614));
#15170=CARTESIAN_POINT('Ctrl Pts',(-2.39787637930257,52.4298989302782,6.77252314615045));
#15171=CARTESIAN_POINT('Ctrl Pts',(0.741361642631027,53.3323569589307,6.61373842692478));
#15172=CARTESIAN_POINT('Ctrl Pts',(3.20189533287493,51.1840972322951,6.45495370769908));
#15173=CARTESIAN_POINT('Ctrl Pts',(2.73114673582125,47.9518160534629,6.29616898847341));
#15174=CARTESIAN_POINT('Ctrl Pts',(-0.239921580162412,46.5946134415093,
6.13738426924771));
#15175=CARTESIAN_POINT('Ctrl Pts',(-2.99134565352125,48.3549859705726,5.97859955002204));
#15176=CARTESIAN_POINT('Ctrl Pts',(-3.00424219532036,51.6213416688123,5.81981483079635));
#15177=CARTESIAN_POINT('Ctrl Pts',(-0.266804635119595,53.4033858527374,
5.66103011157067));
#15178=CARTESIAN_POINT('Ctrl Pts',(2.71488816122889,52.0696865095247,5.50224539234499));
#15179=CARTESIAN_POINT('Ctrl Pts',(3.21114569366885,48.8412233564401,5.3434606731193));
#15180=CARTESIAN_POINT('Ctrl Pts',(0.767652389091321,46.6736010784556,5.18467595389362));
#15181=CARTESIAN_POINT('Ctrl Pts',(-2.37861399671836,47.5512420637604,5.02589123466794));
#15182=CARTESIAN_POINT('Ctrl Pts',(-3.34729856129375,50.6706804881919,4.86710651544225));
#15183=CARTESIAN_POINT('Ctrl Pts',(-1.25158658765491,53.1761220047933,4.70832179621657));
#15184=CARTESIAN_POINT('Ctrl Pts',(1.98993223179098,52.773876292935,4.54953707699088));
#15185=CARTESIAN_POINT('Ctrl Pts',(3.40970096509391,49.832192657113,4.3907523577652));
#15186=CARTESIAN_POINT('Ctrl Pts',(1.70794479033487,47.0441338715863,4.23196763853952));
#15187=CARTESIAN_POINT('Ctrl Pts',(-1.55740662611146,46.9621216982713,4.07318291931384));
#15188=CARTESIAN_POINT('Ctrl Pts',(-3.39697800345581,49.6612369266132,3.91439820008815));
#15189=CARTESIAN_POINT('Ctrl Pts',(-2.12667213392151,52.6704841531413,3.75561348086247));
#15190=CARTESIAN_POINT('Ctrl Pts',(1.09056694327298,53.234947250525,3.59682876163679));
#15191=CARTESIAN_POINT('Ctrl Pts',(3.3094099992828,50.837869581058,3.4380440424111));
#15192=CARTESIAN_POINT('Ctrl Pts',(2.49854286950392,47.6737361464895,3.27925932318542));
#15193=CARTESIAN_POINT('Ctrl Pts',(-0.599698983006457,46.6392588508537,
3.12047460395973));
#15194=CARTESIAN_POINT('Ctrl Pts',(-3.14892632391411,48.6814845426992,2.96168988473405));
#15195=CARTESIAN_POINT('Ctrl Pts',(-2.81536363139498,51.9307893902053,2.80290516550836));
#15196=CARTESIAN_POINT('Ctrl Pts',(0.095617955020209,53.4124883762385,2.64412044628269));
#15197=CARTESIAN_POINT('Ctrl Pts',(2.91906288933533,51.7701107633945,2.485335727057));
#15198=CARTESIAN_POINT('Ctrl Pts',(3.0701539567666,48.5072257144969,2.32655100783131));
#15199=CARTESIAN_POINT('Ctrl Pts',(0.410569817425986,46.610951404296,2.16776628860563));
#15200=CARTESIAN_POINT('Ctrl Pts',(-2.62488425534856,47.8172940318787,2.00898156937995));
#15201=CARTESIAN_POINT('Ctrl Pts',(-3.25730005866627,51.0218700271244,1.85019685015426));
#15202=CARTESIAN_POINT('Ctrl Pts',(-0.907711653352754,53.2909367199938,
1.69141213092858));
#15203=CARTESIAN_POINT('Ctrl Pts',(2.27287214597831,52.547213460909,1.5326274117029));
#15204=CARTESIAN_POINT('Ctrl Pts',(3.37267830997368,49.4715420397218,1.37384269247722));
#15205=CARTESIAN_POINT('Ctrl Pts',(1.38485464191613,46.8796974154137,1.21505797325153));
#15206=CARTESIAN_POINT('Ctrl Pts',(-1.87078343506508,47.1443744644522,1.05627325402585));
#15207=CARTESIAN_POINT('Ctrl Pts',(-3.41374452397723,50.0234556714361,0.897488534800164));
#15208=CARTESIAN_POINT('Ctrl Pts',(-1.83149007927186,52.88081414604,0.738703815574481));
#15209=CARTESIAN_POINT('Ctrl Pts',(1.4274853921914,53.1013281333051,0.579919096348797));
#15210=CARTESIAN_POINT('Ctrl Pts',(3.3795778955967,50.4816519050236,0.421134377123114));
#15211=CARTESIAN_POINT('Ctrl Pts',(2.23780836559748,47.4229621190836,0.262349657897429));
#15212=CARTESIAN_POINT('Ctrl Pts',(-0.952799406850132,46.7196686781745,
0.103564938671747));
#15213=CARTESIAN_POINT('Ctrl Pts',(-3.27090464904435,49.0273058687178,-0.0552197805539384));
#15214=CARTESIAN_POINT('Ctrl Pts',(-2.81936293975441,51.1468332160454,-0.161076260037727));
#15215=CARTESIAN_POINT('Ctrl Pts',(-2.1951971040191,51.8768634390788,-0.214004499779622));
#15216=CARTESIAN_POINT('Ctrl Pts',(-0.698066426161048,47.3888678140614,
10.2140044997796));
#15217=CARTESIAN_POINT('Ctrl Pts',(-1.56641916249635,47.6210153455288,10.1610762600377));
#15218=CARTESIAN_POINT('Ctrl Pts',(-3.03820354494941,49.016276883595,10.0552197805539));
#15219=CARTESIAN_POINT('Ctrl Pts',(-2.47369813414337,52.0247828970048,9.89643506132825));
#15220=CARTESIAN_POINT('Ctrl Pts',(0.359771475385354,53.1737082431722,9.73765034210257));
#15221=CARTESIAN_POINT('Ctrl Pts',(2.86171640707103,51.4200313452195,9.57886562287689));
#15222=CARTESIAN_POINT('Ctrl Pts',(2.74489684265523,48.3648955643612,9.4200809036512));
#15223=CARTESIAN_POINT('Ctrl Pts',(0.114618753812882,46.807400089401,9.26129618442552));
#15224=CARTESIAN_POINT('Ctrl Pts',(-2.62031237460883,48.1723083928789,9.10251146519984));
#15225=CARTESIAN_POINT('Ctrl Pts',(-2.95653166931952,51.210624623909,8.94372674597415));
#15226=CARTESIAN_POINT('Ctrl Pts',(-0.586023824712095,53.1405397176071,
8.78494202674847));
#15227=CARTESIAN_POINT('Ctrl Pts',(2.32094312551941,52.1953902646851,8.62615730752278));
#15228=CARTESIAN_POINT('Ctrl Pts',(3.10314320313993,49.2403731748803,8.46737258829711));
#15229=CARTESIAN_POINT('Ctrl Pts',(1.04445772611147,46.9807940908192,8.30858786907141));
#15230=CARTESIAN_POINT('Ctrl Pts',(-1.97040688608782,47.4852419741422,8.14980314984574));
#15231=CARTESIAN_POINT('Ctrl Pts',(-3.1813988999923,50.2919124074875,7.99101843062005));
#15232=CARTESIAN_POINT('Ctrl Pts',(-1.47987158339412,52.8313402765381,7.83223371139436));
#15233=CARTESIAN_POINT('Ctrl Pts',(1.57645311887049,52.7787236915758,7.67344899216869));
#15234=CARTESIAN_POINT('Ctrl Pts',(3.1895613373074,50.1822310658057,7.514664272943));
#15235=CARTESIAN_POINT('Ctrl Pts',(1.88267868626508,47.418909113619,7.35587955371732));
#15236=CARTESIAN_POINT('Ctrl Pts',(-1.14776512378607,47.0185331272166,7.19709483449163));
#15237=CARTESIAN_POINT('Ctrl Pts',(-3.12744896257627,49.3476408636202,7.03831011526595));
#15238=CARTESIAN_POINT('Ctrl Pts',(-2.2440049191038,52.2739725865498,6.87952539604026));
#15239=CARTESIAN_POINT('Ctrl Pts',(0.693788548591803,53.118519984014,6.72074067681459));
#15240=CARTESIAN_POINT('Ctrl Pts',(2.99643006597223,51.1081138447764,6.5619559575889));
#15241=CARTESIAN_POINT('Ctrl Pts',(2.55588935396233,48.0832477891978,6.40317123836322));
#15242=CARTESIAN_POINT('Ctrl Pts',(-0.224525839084415,46.8131367176962,
6.24438651913753));
#15243=CARTESIAN_POINT('Ctrl Pts',(-2.79939133609292,48.4605463376293,6.08560179991184));
#15244=CARTESIAN_POINT('Ctrl Pts',(-2.81146030824111,51.5173003544999,5.92681708068617));
#15245=CARTESIAN_POINT('Ctrl Pts',(-0.249683811399071,53.184990961616,5.76803236146048));
#15246=CARTESIAN_POINT('Ctrl Pts',(2.54067409029078,51.9368749567177,5.6092476422348));
#15247=CARTESIAN_POINT('Ctrl Pts',(3.00508683214425,48.9155819245998,5.45046292300911));
#15248=CARTESIAN_POINT('Ctrl Pts',(0.718392220779847,46.8870557267768,5.29167820378344));
#15249=CARTESIAN_POINT('Ctrl Pts',(-2.2259786014647,47.708378587801,5.13289348455774));
#15250=CARTESIAN_POINT('Ctrl Pts',(-3.13250278541755,50.627642995961,4.97410876533206));
#15251=CARTESIAN_POINT('Ctrl Pts',(-1.1712724157193,52.9723106094831,4.81532404610638));
#15252=CARTESIAN_POINT('Ctrl Pts',(1.86223850210367,52.5958769601551,4.65653932688069));
#15253=CARTESIAN_POINT('Ctrl Pts',(3.19090083391586,49.8429608356167,4.49775460765502));
#15254=CARTESIAN_POINT('Ctrl Pts',(1.59834616335972,47.23381147184,4.33896988842933));
#15255=CARTESIAN_POINT('Ctrl Pts',(-1.45746801636849,47.1570620105525,4.18018516920365));
#15256=CARTESIAN_POINT('Ctrl Pts',(-3.17899430330907,49.6829753153031,4.02140044997796));
#15257=CARTESIAN_POINT('Ctrl Pts',(-1.99020381994374,52.4991194824566,3.86261573075228));
#15258=CARTESIAN_POINT('Ctrl Pts',(1.02058538398395,53.0273610457479,3.70383101152659));
#15259=CARTESIAN_POINT('Ctrl Pts',(3.09704552821105,50.7841035833584,3.54504629230091));
#15260=CARTESIAN_POINT('Ctrl Pts',(2.33821165184056,47.8230122388839,3.38626157307523));
#15261=CARTESIAN_POINT('Ctrl Pts',(-0.561216366057806,46.8549172360953,
3.22747685384954));
#15262=CARTESIAN_POINT('Ctrl Pts',(-2.94686007241706,48.7660935327458,3.06869213462386));
#15263=CARTESIAN_POINT('Ctrl Pts',(-2.63470206072667,51.8068908500756,2.90990741539818));
#15264=CARTESIAN_POINT('Ctrl Pts',(0.0894821614959184,53.1935093771978,
2.75112269617249));
#15265=CARTESIAN_POINT('Ctrl Pts',(2.73174694883439,51.6565229528518,2.59233797694681));
#15266=CARTESIAN_POINT('Ctrl Pts',(2.87314251929621,48.6030168741415,2.43355325772113));
#15267=CARTESIAN_POINT('Ctrl Pts',(0.384223597968559,46.8284262752304,2.27476853849544));
#15268=CARTESIAN_POINT('Ctrl Pts',(-2.4564457250267,47.9573580307564,2.11598381926976));
#15269=CARTESIAN_POINT('Ctrl Pts',(-3.04827947668019,50.9562967412935,1.95719910004407));
#15270=CARTESIAN_POINT('Ctrl Pts',(-0.849463897652582,53.0797576771966,
1.79841438081839));
#15271=CARTESIAN_POINT('Ctrl Pts',(2.12702219350974,52.3837590568159,1.63962966159271));
#15272=CARTESIAN_POINT('Ctrl Pts',(3.15625391845133,49.5054531281764,1.48084494236703));
#15273=CARTESIAN_POINT('Ctrl Pts',(1.29598867378117,47.0799268847461,1.32206022314134));
#15274=CARTESIAN_POINT('Ctrl Pts',(-1.75073547039358,47.3276196370259,1.16327550391566));
#15275=CARTESIAN_POINT('Ctrl Pts',(-3.19468491807599,50.0219505236124,1.00449078468998));
#15276=CARTESIAN_POINT('Ctrl Pts',(-1.71396356486536,52.6959526231364,0.84570606546429));
#15277=CARTESIAN_POINT('Ctrl Pts',(1.33588381355923,52.9023162523982,0.686921346238609));
#15278=CARTESIAN_POINT('Ctrl Pts',(3.16271075843336,50.4507443559217,0.528136627012924));
#15279=CARTESIAN_POINT('Ctrl Pts',(2.09420845201075,47.588330352887,0.36935190778724));
#15280=CARTESIAN_POINT('Ctrl Pts',(-0.891658375029637,46.9301671737524,
0.210567188561557));
#15281=CARTESIAN_POINT('Ctrl Pts',(-3.0610110620089,49.0897235427894,0.0517824693358723));
#15282=CARTESIAN_POINT('Ctrl Pts',(-2.63844473391409,51.0732410562992,-0.0540740101479162));
#15283=CARTESIAN_POINT('Ctrl Pts',(-2.05433155034207,51.7564253212269,-0.107002249889811));
#15284=CARTESIAN_POINT('Ctrl Pts',(-0.650199997975127,47.5679131979649,
10.3210067496694));
#15285=CARTESIAN_POINT('Ctrl Pts',(-1.4590097705807,47.784142368762,10.2680785099275));
#15286=CARTESIAN_POINT('Ctrl Pts',(-2.82987386979471,49.0837307964915,10.1622220304437));
#15287=CARTESIAN_POINT('Ctrl Pts',(-2.30407660579858,51.8859434950519,10.0034373112181));
#15288=CARTESIAN_POINT('Ctrl Pts',(0.335101938440882,52.95608700827,9.84465259199238));
#15289=CARTESIAN_POINT('Ctrl Pts',(2.66548845833433,51.3226597687329,9.68586787276669));
#15290=CARTESIAN_POINT('Ctrl Pts',(2.55667921368362,48.4770147067691,9.52708315354102));
#15291=CARTESIAN_POINT('Ctrl Pts',(0.106759343672908,47.0263167262997,9.36829843431533));
#15292=CARTESIAN_POINT('Ctrl Pts',(-2.44063750499268,48.2976332413169,9.20951371508965));
#15293=CARTESIAN_POINT('Ctrl Pts',(-2.75380223623798,51.1276120703055,9.05072899586396));
#15294=CARTESIAN_POINT('Ctrl Pts',(-0.545840159849303,52.9251928491371,
8.89194427663828));
#15295=CARTESIAN_POINT('Ctrl Pts',(2.16179601103599,52.0448523122691,8.73315955741259));
#15296=CARTESIAN_POINT('Ctrl Pts',(2.89036061438174,49.2924608007996,8.57437483818692));
#15297=CARTESIAN_POINT('Ctrl Pts',(0.972839239866417,47.187821097726,8.41559011896123));
#15298=CARTESIAN_POINT('Ctrl Pts',(-1.83529604824299,47.6576789800468,8.25680539973555));
#15299=CARTESIAN_POINT('Ctrl Pts',(-2.96325031660503,50.2718959681259,8.09802068050987));
#15300=CARTESIAN_POINT('Ctrl Pts',(-1.37839676063194,52.6371952196527,7.93923596128418));
#15301=CARTESIAN_POINT('Ctrl Pts',(1.46835569837446,52.5881865549271,7.78045124205849));
#15302=CARTESIAN_POINT('Ctrl Pts',(2.9708530554374,50.1697354781399,7.62166652283282));
#15303=CARTESIAN_POINT('Ctrl Pts',(1.75358337275908,47.5958945650376,7.46288180360712));
#15304=CARTESIAN_POINT('Ctrl Pts',(-1.06906284730768,47.2229723676763,7.30409708438145));
#15305=CARTESIAN_POINT('Ctrl Pts',(-2.9129997274289,49.3923731420721,7.14531236515576));
#15306=CARTESIAN_POINT('Ctrl Pts',(-2.09013345890504,52.1180462428214,6.98652764593008));
#15307=CARTESIAN_POINT('Ctrl Pts',(0.646215454552581,52.9046830090973,6.82774292670439));
#15308=CARTESIAN_POINT('Ctrl Pts',(2.79096479906952,51.0321304572577,6.66895820747871));
#15309=CARTESIAN_POINT('Ctrl Pts',(2.38063197210341,48.2146795249326,6.51017348825303));
#15310=CARTESIAN_POINT('Ctrl Pts',(-0.20913009800642,47.031659993883,6.35138876902734));
#15311=CARTESIAN_POINT('Ctrl Pts',(-2.60743701866458,48.5661067046858,6.19260404980165));
#15312=CARTESIAN_POINT('Ctrl Pts',(-2.61867842116187,51.4132590401875,6.03381933057598));
#15313=CARTESIAN_POINT('Ctrl Pts',(-0.232562987678543,52.9665960704945,
5.87503461135029));
#15314=CARTESIAN_POINT('Ctrl Pts',(2.36646001935266,51.8040634039108,5.71624989212461));
#15315=CARTESIAN_POINT('Ctrl Pts',(2.79902797061965,48.9899404927595,5.55746517289893));
#15316=CARTESIAN_POINT('Ctrl Pts',(0.66913205246837,47.1005103750979,5.39868045367324));
#15317=CARTESIAN_POINT('Ctrl Pts',(-2.07334320621103,47.8655151118416,5.23989573444756));
#15318=CARTESIAN_POINT('Ctrl Pts',(-2.91770700954136,50.5846055037301,5.08111101522187));
#15319=CARTESIAN_POINT('Ctrl Pts',(-1.09095824378368,52.7684992141729,4.92232629599619));
#15320=CARTESIAN_POINT('Ctrl Pts',(1.73454477241634,52.4178776273751,4.7635415767705));
#15321=CARTESIAN_POINT('Ctrl Pts',(2.97210070273781,49.8537290141204,4.60475685754483));
#15322=CARTESIAN_POINT('Ctrl Pts',(1.48874753638457,47.4234890720937,4.44597213831914));
#15323=CARTESIAN_POINT('Ctrl Pts',(-1.35752940662552,47.3520023228338,4.28718741909346));
#15324=CARTESIAN_POINT('Ctrl Pts',(-2.96101060316233,49.7047137039929,4.12840269986777));
#15325=CARTESIAN_POINT('Ctrl Pts',(-1.85373550596597,52.327754811772,3.96961798064209));
#15326=CARTESIAN_POINT('Ctrl Pts',(0.950603824694923,52.8197748409707,3.8108332614164));
#15327=CARTESIAN_POINT('Ctrl Pts',(2.88468105713929,50.7303375856587,3.65204854219073));
#15328=CARTESIAN_POINT('Ctrl Pts',(2.1778804341772,47.9722883312785,3.49326382296504));
#15329=CARTESIAN_POINT('Ctrl Pts',(-0.522733749109153,47.0705756213368,
3.33447910373936));
#15330=CARTESIAN_POINT('Ctrl Pts',(-2.74479382092,48.8507025227925,3.17569438451367));
#15331=CARTESIAN_POINT('Ctrl Pts',(-2.45404049005835,51.6829923099458,3.01690966528799));
#15332=CARTESIAN_POINT('Ctrl Pts',(0.0833463679716227,52.974530378157,2.85812494606231));
#15333=CARTESIAN_POINT('Ctrl Pts',(2.54443100833344,51.5429351423091,2.69934022683662));
#15334=CARTESIAN_POINT('Ctrl Pts',(2.67613108182581,48.6988080337859,2.54055550761094));
#15335=CARTESIAN_POINT('Ctrl Pts',(0.357877378511138,47.0459011461649,2.38177078838525));
#15336=CARTESIAN_POINT('Ctrl Pts',(-2.28800719470483,48.0974220296341,2.22298606915957));
#15337=CARTESIAN_POINT('Ctrl Pts',(-2.8392588946941,50.8907234554627,2.06420134993389));
#15338=CARTESIAN_POINT('Ctrl Pts',(-0.791216141952413,52.8685786343994,
1.9054166307082));
#15339=CARTESIAN_POINT('Ctrl Pts',(1.98117224104117,52.2203046527227,1.74663191148252));
#15340=CARTESIAN_POINT('Ctrl Pts',(2.93982952692898,49.539364216631,1.58784719225684));
#15341=CARTESIAN_POINT('Ctrl Pts',(1.20712270564621,47.2801563540783,1.42906247303115));
#15342=CARTESIAN_POINT('Ctrl Pts',(-1.63068750572208,47.5108648095996,1.27027775380547));
#15343=CARTESIAN_POINT('Ctrl Pts',(-2.97562531217475,50.0204453757886,1.11149303457979));
#15344=CARTESIAN_POINT('Ctrl Pts',(-1.59643705045885,52.5110911002329,0.952708315354101));
#15345=CARTESIAN_POINT('Ctrl Pts',(1.24428223492706,52.7033043714913,0.79392359612842));
#15346=CARTESIAN_POINT('Ctrl Pts',(2.94584362127002,50.4198368068199,0.635138876902735));
#15347=CARTESIAN_POINT('Ctrl Pts',(1.95060853842403,47.7536985866904,0.476354157677051));
#15348=CARTESIAN_POINT('Ctrl Pts',(-0.830517343209144,47.1406656693304,
0.317569438451368));
#15349=CARTESIAN_POINT('Ctrl Pts',(-2.85111747497345,49.1521412168609,0.158784719225683));
#15350=CARTESIAN_POINT('Ctrl Pts',(-2.45752652807377,50.999648896553,0.0529282397418946));
#15351=CARTESIAN_POINT('Ctrl Pts',(-1.91346599666504,51.635987203375,0.));
#15352=CARTESIAN_POINT('Ctrl Pts',(-1.91346599666504,51.635987203375,0.));
#15353=CARTESIAN_POINT('Ctrl Pts',(-1.97508250372926,51.5780828168137,-7.88547235160471E-17));
#15354=CARTESIAN_POINT('Ctrl Pts',(-2.03332802563557,51.517028168085,-1.95903716127754E-15));
#15355=CARTESIAN_POINT('Ctrl Pts',(-2.0882055508515,51.4532079963186,-1.60982338570648E-15));
#15356=CARTESIAN_POINT('Ctrl Pts',(-2.14453544714772,51.3876987802404,-1.25136742972581E-15));
#15357=CARTESIAN_POINT('Ctrl Pts',(-2.1973171511753,51.3192752892963,-2.54643214235558E-15));
#15358=CARTESIAN_POINT('Ctrl Pts',(-2.24652834894968,51.2483050710386,-2.88657986402541E-15));
#15359=CARTESIAN_POINT('Ctrl Pts',(-2.29743052792617,51.1748961942964,-3.23841564510647E-15));
#15360=CARTESIAN_POINT('Ctrl Pts',(-2.34451318991709,51.0987620412396,1.26930694503224E-15));
#15361=CARTESIAN_POINT('Ctrl Pts',(-2.38771671870761,51.0202653810526,9.99200722162641E-16));
#15362=CARTESIAN_POINT('Ctrl Pts',(-2.40661826255346,50.9859230922208,8.81029249657191E-16));
#15363=CARTESIAN_POINT('Ctrl Pts',(-2.42477682213031,50.9511280985978,-4.72647997039093E-15));
#15364=CARTESIAN_POINT('Ctrl Pts',(-2.44218496027157,50.9159086901715,-5.16253706450698E-15));
#15365=CARTESIAN_POINT('Ctrl Pts',(-2.4516917365468,50.8966749827102,-5.40067265392762E-15));
#15366=CARTESIAN_POINT('Ctrl Pts',(-2.4609746819567,50.8773146792715,1.38692847400875E-15));
#15367=CARTESIAN_POINT('Ctrl Pts',(-2.47003238168185,50.857832258915,1.60982338570648E-15));
#15368=CARTESIAN_POINT('Ctrl Pts',(-2.47868101112295,50.8392297174981,1.82265175870151E-15));
#15369=CARTESIAN_POINT('Ctrl Pts',(-2.48712676984399,50.8205098452481,-2.92077872961859E-16));
#15370=CARTESIAN_POINT('Ctrl Pts',(-2.49535433119684,50.801709305486,-2.22044604925031E-16));
#15371=CARTESIAN_POINT('Ctrl Pts',(-2.53191983250978,50.7181546369918,8.92021235434719E-17));
#15372=CARTESIAN_POINT('Ctrl Pts',(-2.56422492917263,50.6329165377822,5.94993583842564E-16));
#15373=CARTESIAN_POINT('Ctrl Pts',(-2.59224521232009,50.546393762837,5.82867087928207E-16));
#15374=CARTESIAN_POINT('Ctrl Pts',(-2.62072727043851,50.4584450903848,5.70540747056209E-16));
#15375=CARTESIAN_POINT('Ctrl Pts',(-2.64478261577045,50.3691682946478,1.3966825979773E-15));
#15376=CARTESIAN_POINT('Ctrl Pts',(-2.66434650648327,50.2789450457094,9.43689570931383E-16));
#15377=CARTESIAN_POINT('Ctrl Pts',(-2.68357149093349,50.1902847386492,4.98543764872047E-16));
#15378=CARTESIAN_POINT('Ctrl Pts',(-2.6984595431006,50.1007095761311,-1.44477158663301E-15));
#15379=CARTESIAN_POINT('Ctrl Pts',(-2.70890652948763,50.0105588921822,-1.74860126378462E-15));
#15380=CARTESIAN_POINT('Ctrl Pts',(-2.71303741983049,49.9749120007313,-1.86873993657737E-15));
#15381=CARTESIAN_POINT('Ctrl Pts',(-2.71647344141028,49.9391749440761,-4.57020580419667E-16));
#15382=CARTESIAN_POINT('Ctrl Pts',(-2.71920612755143,49.9033681666514,-7.21644966006352E-16));
#15383=CARTESIAN_POINT('Ctrl Pts',(-2.72082363900511,49.8821736826851,-8.78279483290925E-16));
#15384=CARTESIAN_POINT('Ctrl Pts',(-2.7221947068849,49.8609547672148,-1.34276899995115E-15));
#15385=CARTESIAN_POINT('Ctrl Pts',(-2.72331737293965,49.8397156372056,-1.41553435639707E-15));
#15386=CARTESIAN_POINT('Ctrl Pts',(-2.72406463156244,49.8255786434197,-1.46396776169497E-15));
#15387=CARTESIAN_POINT('Ctrl Pts',(-2.7247017593876,49.8114326986645,-2.92576848619345E-16));
#15388=CARTESIAN_POINT('Ctrl Pts',(-2.72522782764266,49.797293600135,-4.16333634234434E-16));
#15389=CARTESIAN_POINT('Ctrl Pts',(-2.72876903784861,49.7021167489681,-1.24939814261499E-15));
#15390=CARTESIAN_POINT('Ctrl Pts',(-2.72729103062767,49.6070885424556,8.33615584934857E-16));
#15391=CARTESIAN_POINT('Ctrl Pts',(-2.72073501618782,49.5126075692422,6.93889390390723E-16));
#15392=CARTESIAN_POINT('Ctrl Pts',(-2.71420165583577,49.4184530718599,5.54646015021133E-16));
#15393=CARTESIAN_POINT('Ctrl Pts',(-2.70262568072403,49.3248410792282,-1.79204710018197E-16));
#15394=CARTESIAN_POINT('Ctrl Pts',(-2.68590091265149,49.2321481599992,2.77555756156289E-16));
#15395=CARTESIAN_POINT('Ctrl Pts',(-2.68396405390562,49.2214135961171,3.30452184964298E-16));
#15396=CARTESIAN_POINT('Ctrl Pts',(-2.68195808574165,49.2106913478966,-6.33066629083406E-15));
#15397=CARTESIAN_POINT('Ctrl Pts',(-2.67988279801038,49.1999819937366,-6.41153796721028E-15));
#15398=CARTESIAN_POINT('Ctrl Pts',(-2.66233852493469,49.1094461942822,-7.09521895903373E-15));
#15399=CARTESIAN_POINT('Ctrl Pts',(-2.63984447556841,49.0198316064943,-8.66493849292325E-16));
#15400=CARTESIAN_POINT('Ctrl Pts',(-2.61267603168784,48.9313762482598,-1.11022302462516E-15));
#15401=CARTESIAN_POINT('Ctrl Pts',(-2.60192825571706,48.8963835052856,-1.20664174428155E-15));
#15402=CARTESIAN_POINT('Ctrl Pts',(-2.59044836827368,48.861572229629,-5.47531613863234E-16));
#15403=CARTESIAN_POINT('Ctrl Pts',(-2.57825122455276,48.8269574989795,-3.60822483003176E-16));
#15404=CARTESIAN_POINT('Ctrl Pts',(-2.57231287966207,48.8101048477688,-2.69920609691125E-16));
#15405=CARTESIAN_POINT('Ctrl Pts',(-2.56620450114377,48.7932987890619,-9.87740507932057E-16));
#15406=CARTESIAN_POINT('Ctrl Pts',(-2.55992770321574,48.7765410907625,-9.15933995315754E-16));
#15407=CARTESIAN_POINT('Ctrl Pts',(-2.55466778336413,48.762498237868,-8.55760558873183E-16));
#15408=CARTESIAN_POINT('Ctrl Pts',(-2.54929245582117,48.7484970704423,-1.04336745179747E-15));
#15409=CARTESIAN_POINT('Ctrl Pts',(-2.54380502947758,48.7345433945498,-9.43689570931383E-16));
#15410=CARTESIAN_POINT('Ctrl Pts',(-2.50958084575905,48.6475165922947,-3.22014874300647E-16));
#15411=CARTESIAN_POINT('Ctrl Pts',(-2.47097808219571,48.5622772719038,-2.76096825153635E-15));
#15412=CARTESIAN_POINT('Ctrl Pts',(-2.42832930579416,48.4790573924985,-2.45636844198316E-15));
#15413=CARTESIAN_POINT('Ctrl Pts',(-2.38409930402159,48.3927520931635,-2.14047543746612E-15));
#15414=CARTESIAN_POINT('Ctrl Pts',(-2.3355175823713,48.3086180283362,-4.37014208287737E-16));
#15415=CARTESIAN_POINT('Ctrl Pts',(-2.28289912148411,48.2269174441202,-1.9151347174784E-15));
#15416=CARTESIAN_POINT('Ctrl Pts',(-2.2297022750075,48.1443188016988,-3.40950282470803E-15));
#15417=CARTESIAN_POINT('Ctrl Pts',(-2.17237903905252,48.0642066138853,1.84196985151739E-15));
#15418=CARTESIAN_POINT('Ctrl Pts',(-2.11120327391795,47.9868672202785,1.81799020282369E-15));
#15419=CARTESIAN_POINT('Ctrl Pts',(-2.08739408923495,47.9567672631859,1.80865748940155E-15));
#15420=CARTESIAN_POINT('Ctrl Pts',(-2.06300084281701,47.9270875343801,-2.70289509530768E-15));
#15421=CARTESIAN_POINT('Ctrl Pts',(-2.03803781529234,47.8978459523877,-2.88657986402541E-15));
#15422=CARTESIAN_POINT('Ctrl Pts',(-2.01823971473763,47.8746545434093,-3.03225969063487E-15));
#15423=CARTESIAN_POINT('Ctrl Pts',(-1.99808319977527,47.8517387409254,-3.30551557830788E-15));
#15424=CARTESIAN_POINT('Ctrl Pts',(-1.97757497212805,47.8291078145036,-3.4555691641458E-15));
#15425=CARTESIAN_POINT('Ctrl Pts',(-1.96583741766514,47.8161553675154,-3.54144992217255E-15));
#15426=CARTESIAN_POINT('Ctrl Pts',(-1.95398941490868,47.8033015714534,1.65071552113353E-15));
#15427=CARTESIAN_POINT('Ctrl Pts',(-1.9420381151495,47.7905538223288,1.48492329543615E-15));
#15428=CARTESIAN_POINT('Ctrl Pts',(-1.87298185596159,47.7168955688038,5.26952937416942E-16));
#15429=CARTESIAN_POINT('Ctrl Pts',(-1.80042495380938,47.6467145489693,-8.25147557761074E-16));
#15430=CARTESIAN_POINT('Ctrl Pts',(-1.72467948086462,47.5802997238268,-1.94289029309402E-16));
#15431=CARTESIAN_POINT('Ctrl Pts',(-1.66042054073069,47.5239564717893,3.4090203672718E-16));
#15432=CARTESIAN_POINT('Ctrl Pts',(-1.59386571260425,47.4703237412601,1.07379577703767E-16));
#15433=CARTESIAN_POINT('Ctrl Pts',(-1.52518066669226,47.4195928883885,-7.35522753814166E-16));
#15434=CARTESIAN_POINT('Ctrl Pts',(-1.50256447612399,47.4028885443642,-1.01306846273714E-15));
#15435=CARTESIAN_POINT('Ctrl Pts',(-1.47971715840407,47.3864989618495,-1.85072163263063E-15));
#15436=CARTESIAN_POINT('Ctrl Pts',(-1.45664416191384,47.3704314082844,-2.14411821630733E-15));
#15437=CARTESIAN_POINT('Ctrl Pts',(-1.43995378600627,47.3588085785826,-2.35635329698423E-15));
#15438=CARTESIAN_POINT('Ctrl Pts',(-1.42314427660525,47.347353683751,-3.1683259339951E-15));
#15439=CARTESIAN_POINT('Ctrl Pts',(-1.4062324772292,47.3360791105664,-3.08086889333481E-15));
#15440=CARTESIAN_POINT('Ctrl Pts',(-1.31987495994381,47.278507226758,-2.634282889527E-15));
#15441=CARTESIAN_POINT('Ctrl Pts',(-1.23076834239895,47.2255739050535,4.26208680824903E-15));
#15442=CARTESIAN_POINT('Ctrl Pts',(-1.13922130482109,47.1776007437286,2.75127143289922E-15));
#15443=CARTESIAN_POINT('Ctrl Pts',(-1.04767426724323,47.1296275824037,1.2404560575494E-15));
#15444=CARTESIAN_POINT('Ctrl Pts',(-0.953686164033146,47.0866136704993,
-2.39983802697838E-15));
#15445=CARTESIAN_POINT('Ctrl Pts',(-0.857527633333973,47.0489213548329,
-3.9118014383277E-15));
#15446=CARTESIAN_POINT('Ctrl Pts',(-0.836959291797765,47.0408589560391,
-4.28706450102705E-15));
#15447=CARTESIAN_POINT('Ctrl Pts',(-0.816291527885438,47.0330402152543,
-8.74346376558217E-17));
#15448=CARTESIAN_POINT('Ctrl Pts',(-0.795528245027205,47.0254639548254,
-5.55111512312578E-17));
#15449=CARTESIAN_POINT('Ctrl Pts',(-2.51421069693398,50.0014124180709,9.11258330249199));
#15450=CARTESIAN_POINT('Ctrl Pts',(-2.51589016857918,50.3285491477533,9.09196520028265));
#15451=CARTESIAN_POINT('Ctrl Pts',(-2.45663359423571,50.6551027847351,9.07134709807331));
#15452=CARTESIAN_POINT('Ctrl Pts',(-2.33361443496565,50.9555457286126,9.05072899586397));
#15453=CARTESIAN_POINT('Ctrl Pts',(-2.01781487744175,51.7268056632493,8.99780075612207));
#15454=CARTESIAN_POINT('Ctrl Pts',(-1.28182751864553,52.3259992561932,8.94487251638018));
#15455=CARTESIAN_POINT('Ctrl Pts',(-0.462561144099867,52.4788726298538,
8.89194427663828));
#15456=CARTESIAN_POINT('Ctrl Pts',(0.356705230445793,52.6317460035144,8.83901603689639));
#15457=CARTESIAN_POINT('Ctrl Pts',(1.25925062074089,52.3382991578918,8.78608779715449));
#15458=CARTESIAN_POINT('Ctrl Pts',(1.83195074977939,51.7328438165022,8.7331595574126));
#15459=CARTESIAN_POINT('Ctrl Pts',(2.4046508788179,51.1273884751126,8.6802313176707));
#15460=CARTESIAN_POINT('Ctrl Pts',(2.64750574659982,50.2099246379561,8.62730307792881));
#15461=CARTESIAN_POINT('Ctrl Pts',(2.44934628473822,49.4004194355323,8.57437483818692));
#15462=CARTESIAN_POINT('Ctrl Pts',(2.25118682287662,48.5909142331084,8.52144659844502));
#15463=CARTESIAN_POINT('Ctrl Pts',(1.61201303137152,47.8893676654172,8.46851835870313));
#15464=CARTESIAN_POINT('Ctrl Pts',(0.824403587600737,47.6169040286251,8.41559011896123));
#15465=CARTESIAN_POINT('Ctrl Pts',(0.0367941438299503,47.3444403918329,
8.36266187921934));
#15466=CARTESIAN_POINT('Ctrl Pts',(-0.899250952206518,47.5010596859399,
8.30973363947744));
#15467=CARTESIAN_POINT('Ctrl Pts',(-1.55526587828509,48.0150721643398,8.25680539973555));
#15468=CARTESIAN_POINT('Ctrl Pts',(-2.15111571146493,48.4819430194556,8.20873136732103));
#15469=CARTESIAN_POINT('Ctrl Pts',(-2.51594477493577,49.2436579927481,8.16065733490651));
#15470=CARTESIAN_POINT('Ctrl Pts',(-2.52079116141582,50.0013273547755,8.11258330249199));
#15471=CARTESIAN_POINT('Ctrl Pts',(-0.79379928253289,47.0307770462543,10.));
#15472=CARTESIAN_POINT('Ctrl Pts',(-0.88685746467595,47.0648181449704,10.));
#15473=CARTESIAN_POINT('Ctrl Pts',(-0.977848397661759,47.1036281235935,
10.));
#15474=CARTESIAN_POINT('Ctrl Pts',(-1.06656423869436,47.1468784092156,10.));
#15475=CARTESIAN_POINT('Ctrl Pts',(-1.15724789156607,47.1910880322357,10.));
#15476=CARTESIAN_POINT('Ctrl Pts',(-1.24555507223239,47.2399377454417,10.));
#15477=CARTESIAN_POINT('Ctrl Pts',(-1.33123485996843,47.2931221720949,10.));
#15478=CARTESIAN_POINT('Ctrl Pts',(-1.41418373231515,47.3446114245062,10.));
#15479=CARTESIAN_POINT('Ctrl Pts',(-1.49467035617305,47.4001643315653,10.));
#15480=CARTESIAN_POINT('Ctrl Pts',(-1.57243333752743,47.4595344816828,10.));
#15481=CARTESIAN_POINT('Ctrl Pts',(-1.64047594621252,47.5114833630356,10.));
#15482=CARTESIAN_POINT('Ctrl Pts',(-1.70643296936772,47.5663555378622,10.));
#15483=CARTESIAN_POINT('Ctrl Pts',(-1.77010402938273,47.6239989062131,10.));
#15484=CARTESIAN_POINT('Ctrl Pts',(-1.78344377116941,47.6360757846149,10.));
#15485=CARTESIAN_POINT('Ctrl Pts',(-1.79668493788908,47.648276201783,10.));
#15486=CARTESIAN_POINT('Ctrl Pts',(-1.80980851672957,47.6605824648445,10.));
#15487=CARTESIAN_POINT('Ctrl Pts',(-1.88223677518892,47.7285000056708,10.));
#15488=CARTESIAN_POINT('Ctrl Pts',(-1.95119933213202,47.7997385749445,10.));
#15489=CARTESIAN_POINT('Ctrl Pts',(-2.01645680990078,47.8740071988597,10.));
#15490=CARTESIAN_POINT('Ctrl Pts',(-2.08135213335938,47.9478636600132,10.));
#15491=CARTESIAN_POINT('Ctrl Pts',(-2.14258387218845,48.0247174355525,10.));
#15492=CARTESIAN_POINT('Ctrl Pts',(-2.19987299961007,48.1043091145767,10.));
#15493=CARTESIAN_POINT('Ctrl Pts',(-2.25572878425838,48.1819094531306,10.));
#15494=CARTESIAN_POINT('Ctrl Pts',(-2.30783704358244,48.2621131469488,10.));
#15495=CARTESIAN_POINT('Ctrl Pts',(-2.35589231127005,48.3446938995333,10.));
#15496=CARTESIAN_POINT('Ctrl Pts',(-2.37661982896018,48.3803131790093,10.));
#15497=CARTESIAN_POINT('Ctrl Pts',(-2.39659269249857,48.4163748099892,10.));
#15498=CARTESIAN_POINT('Ctrl Pts',(-2.41578340672494,48.4528609664052,10.));
#15499=CARTESIAN_POINT('Ctrl Pts',(-2.42944475906872,48.4788344779999,10.));
#15500=CARTESIAN_POINT('Ctrl Pts',(-2.44270970882733,48.5050231267819,10.));
#15501=CARTESIAN_POINT('Ctrl Pts',(-2.45556774116037,48.531420485817,10.));
#15502=CARTESIAN_POINT('Ctrl Pts',(-2.46118157523555,48.542945607998,10.));
#15503=CARTESIAN_POINT('Ctrl Pts',(-2.46671692321559,48.5545087352933,10.));
#15504=CARTESIAN_POINT('Ctrl Pts',(-2.47216920778115,48.5661010414056,10.));
#15505=CARTESIAN_POINT('Ctrl Pts',(-2.51239820905703,48.65163342545,10.));
#15506=CARTESIAN_POINT('Ctrl Pts',(-2.54817121352112,48.7388794985857,10.));
#15507=CARTESIAN_POINT('Ctrl Pts',(-2.57923722849636,48.8276021287986,10.));
#15508=CARTESIAN_POINT('Ctrl Pts',(-2.60961658325033,48.914363699605,10.));
#15509=CARTESIAN_POINT('Ctrl Pts',(-2.63549494599023,49.0025379497205,10.));
#15510=CARTESIAN_POINT('Ctrl Pts',(-2.65658848539868,49.0919119517006,10.));
#15511=CARTESIAN_POINT('Ctrl Pts',(-2.66032107555693,49.1077270557348,10.));
#15512=CARTESIAN_POINT('Ctrl Pts',(-2.66390370811112,49.1235797355961,10.));
#15513=CARTESIAN_POINT('Ctrl Pts',(-2.66733463762423,49.139468817129,10.));
#15514=CARTESIAN_POINT('Ctrl Pts',(-2.68744534109363,49.2326041047786,10.));
#15515=CARTESIAN_POINT('Ctrl Pts',(-2.70234787596852,49.3269911317428,10.));
#15516=CARTESIAN_POINT('Ctrl Pts',(-2.7121207670544,49.422220824992,10.));
#15517=CARTESIAN_POINT('Ctrl Pts',(-2.71539839184387,49.4541588871832,10.));
#15518=CARTESIAN_POINT('Ctrl Pts',(-2.71809862149407,49.4861916106476,10.));
#15519=CARTESIAN_POINT('Ctrl Pts',(-2.72022319348791,49.5183030945014,10.));
#15520=CARTESIAN_POINT('Ctrl Pts',(-2.721411705215,49.5362666538656,10.));
#15521=CARTESIAN_POINT('Ctrl Pts',(-2.72242005876359,49.5542548554015,10.));
#15522=CARTESIAN_POINT('Ctrl Pts',(-2.72324847895075,49.5722648704493,10.));
#15523=CARTESIAN_POINT('Ctrl Pts',(-2.72382264730573,49.5847474015046,10.));
#15524=CARTESIAN_POINT('Ctrl Pts',(-2.72431026565451,49.5972388825475,10.));
#15525=CARTESIAN_POINT('Ctrl Pts',(-2.72471128394146,49.6097288907187,10.));
#15526=CARTESIAN_POINT('Ctrl Pts',(-2.72770346772776,49.7029226456101,10.));
#15527=CARTESIAN_POINT('Ctrl Pts',(-2.72588593808555,49.7961815023849,10.));
#15528=CARTESIAN_POINT('Ctrl Pts',(-2.71939783159665,49.8891301579573,10.));
#15529=CARTESIAN_POINT('Ctrl Pts',(-2.71289677354566,49.9822643576922,10.));
#15530=CARTESIAN_POINT('Ctrl Pts',(-2.70170608968587,50.0750880985227,10.));
#15531=CARTESIAN_POINT('Ctrl Pts',(-2.68591470530057,50.1672118275468,10.));
#15532=CARTESIAN_POINT('Ctrl Pts',(-2.67034661567951,50.258032900271,10.));
#15533=CARTESIAN_POINT('Ctrl Pts',(-2.65030654814482,50.3481744652969,10.));
#15534=CARTESIAN_POINT('Ctrl Pts',(-2.62583666370597,50.4372381109382,10.));
#15535=CARTESIAN_POINT('Ctrl Pts',(-2.61632323783499,50.4718643631678,10.));
#15536=CARTESIAN_POINT('Ctrl Pts',(-2.60613981410898,50.5063273483527,10.));
#15537=CARTESIAN_POINT('Ctrl Pts',(-2.59528730377686,50.540602191635,10.));
#15538=CARTESIAN_POINT('Ctrl Pts',(-2.58948288707972,50.5589339385351,10.));
#15539=CARTESIAN_POINT('Ctrl Pts',(-2.58348705736666,50.5772118500355,10.));
#15540=CARTESIAN_POINT('Ctrl Pts',(-2.57729985835685,50.5954320059774,10.));
#15541=CARTESIAN_POINT('Ctrl Pts',(-2.5718499952794,50.6114808440665,10.));
#15542=CARTESIAN_POINT('Ctrl Pts',(-2.56625117625606,50.6274859495329,10.));
#15543=CARTESIAN_POINT('Ctrl Pts',(-2.56050955613592,50.6434282233615,10.));
#15544=CARTESIAN_POINT('Ctrl Pts',(-2.52808295054336,50.733464452661,10.));
#15545=CARTESIAN_POINT('Ctrl Pts',(-2.49106530982848,50.8216219280263,10.));
#15546=CARTESIAN_POINT('Ctrl Pts',(-2.44952970456379,50.9074558899223,10.));
#15547=CARTESIAN_POINT('Ctrl Pts',(-2.41837800061528,50.9718313613443,10.));
#15548=CARTESIAN_POINT('Ctrl Pts',(-2.38468379325917,51.034899319489,10.));
#15549=CARTESIAN_POINT('Ctrl Pts',(-2.34846054129087,51.0964549719667,10.));
#15550=CARTESIAN_POINT('Ctrl Pts',(-2.33352933951851,51.1218281733618,10.));
#15551=CARTESIAN_POINT('Ctrl Pts',(-2.31816826890919,51.1469442216261,10.));
#15552=CARTESIAN_POINT('Ctrl Pts',(-2.30237761435193,51.1717878682362,10.));
#15553=CARTESIAN_POINT('Ctrl Pts',(-2.29294420526028,51.1866295760927,10.));
#15554=CARTESIAN_POINT('Ctrl Pts',(-2.28336215805488,51.2013666481012,10.));
#15555=CARTESIAN_POINT('Ctrl Pts',(-2.27363351537069,51.2159937552642,10.));
#15556=CARTESIAN_POINT('Ctrl Pts',(-2.22610549637866,51.2874525856076,10.));
#15557=CARTESIAN_POINT('Ctrl Pts',(-2.17506897708167,51.3563092144139,10.));
#15558=CARTESIAN_POINT('Ctrl Pts',(-2.12055836507602,51.422210815454,10.));
#15559=CARTESIAN_POINT('Ctrl Pts',(-2.06896996837888,51.484579550868,10.));
#15560=CARTESIAN_POINT('Ctrl Pts',(-2.01426948381755,51.5443018134259,10.));
#15561=CARTESIAN_POINT('Ctrl Pts',(-1.95646228443515,51.6010426460372,10.));
#15562=CARTESIAN_POINT('Ctrl Pts',(-1.94349623175226,51.6137695145375,10.));
#15563=CARTESIAN_POINT('Ctrl Pts',(-1.93037379547304,51.6263462293885,10.));
#15564=CARTESIAN_POINT('Ctrl Pts',(-1.91709820558804,51.6387714616175,10.));
#15565=CARTESIAN_POINT('Origin',(0.,50.,10.));
#15566=CARTESIAN_POINT('',(-6.,50.,10.));
#15567=CARTESIAN_POINT('Origin',(0.,50.,10.));
#15568=CARTESIAN_POINT('Origin',(0.,50.,5.));
#15569=CARTESIAN_POINT('Origin',(-15.,0.,2.));
#15570=CARTESIAN_POINT('',(-18.,3.67394039744206E-16,4.));
#15571=CARTESIAN_POINT('Origin',(-15.,0.,4.));
#15572=CARTESIAN_POINT('',(-18.,3.67394039744206E-16,0.));
#15573=CARTESIAN_POINT('',(-18.,3.67394039744206E-16,2.));
#15574=CARTESIAN_POINT('Origin',(-15.,0.,0.));
#15575=CARTESIAN_POINT('Origin',(15.,0.,2.));
#15576=CARTESIAN_POINT('',(12.,3.67394039744206E-16,4.));
#15577=CARTESIAN_POINT('Origin',(15.,0.,4.));
#15578=CARTESIAN_POINT('',(12.,3.67394039744206E-16,0.));
#15579=CARTESIAN_POINT('',(12.,3.67394039744206E-16,2.));
#15580=CARTESIAN_POINT('Origin',(15.,0.,0.));
#15581=CARTESIAN_POINT('Origin',(0.,0.,2.));
#15582=CARTESIAN_POINT('',(-5.,6.12323399573677E-16,4.));
#15583=CARTESIAN_POINT('Origin',(0.,0.,4.));
#15584=CARTESIAN_POINT('',(-5.,6.12323399573677E-16,0.));
#15585=CARTESIAN_POINT('',(-5.,6.12323399573677E-16,2.));
#15586=CARTESIAN_POINT('Origin',(0.,0.,0.));
#15587=CARTESIAN_POINT('Origin',(0.,50.,0.));
#15588=CARTESIAN_POINT('',(-6.,50.,4.));
#15589=CARTESIAN_POINT('',(-6.,50.,0.));
#15590=CARTESIAN_POINT('Origin',(0.,50.,4.));
#15591=CARTESIAN_POINT('Origin',(0.,50.,0.));
#15592=CARTESIAN_POINT('',(10.,50.,0.));
#15593=CARTESIAN_POINT('',(10.,50.,4.));
#15594=CARTESIAN_POINT('',(10.,50.,0.));
#15595=CARTESIAN_POINT('',(-10.,50.,0.));
#15596=CARTESIAN_POINT('Origin',(0.,50.,0.));
#15597=CARTESIAN_POINT('',(-10.,50.,4.));
#15598=CARTESIAN_POINT('',(-10.,50.,0.));
#15599=CARTESIAN_POINT('Origin',(0.,50.,4.));
#15600=CARTESIAN_POINT('Origin',(0.,0.,4.));
#15601=CARTESIAN_POINT('',(-10.,6.,4.));
#15602=CARTESIAN_POINT('',(-10.,50.,4.));
#15603=CARTESIAN_POINT('',(-15.,6.,4.));
#15604=CARTESIAN_POINT('',(15.,6.,4.));
#15605=CARTESIAN_POINT('',(-15.,-6.,4.));
#15606=CARTESIAN_POINT('Origin',(-15.,0.,4.));
#15607=CARTESIAN_POINT('',(-5.29150262212918,-6.,4.));
#15608=CARTESIAN_POINT('',(-15.,-6.,4.));
#15609=CARTESIAN_POINT('',(5.29150262212918,-6.,4.));
#15610=CARTESIAN_POINT('Origin',(0.,0.,4.));
#15611=CARTESIAN_POINT('',(15.,-6.,4.));
#15612=CARTESIAN_POINT('',(-15.,-6.,4.));
#15613=CARTESIAN_POINT('',(15.,6.,4.));
#15614=CARTESIAN_POINT('Origin',(15.,0.,4.));
#15615=CARTESIAN_POINT('',(10.,6.,4.));
#15616=CARTESIAN_POINT('',(15.,6.,4.));
#15617=CARTESIAN_POINT('',(10.,0.,4.));
#15618=CARTESIAN_POINT('Origin',(10.,0.,0.));
#15619=CARTESIAN_POINT('',(10.,6.,0.));
#15620=CARTESIAN_POINT('',(10.,6.,0.));
#15621=CARTESIAN_POINT('',(10.,0.,0.));
#15622=CARTESIAN_POINT('Origin',(-10.,50.,0.));
#15623=CARTESIAN_POINT('',(-10.,6.,0.));
#15624=CARTESIAN_POINT('',(-10.,6.,0.));
#15625=CARTESIAN_POINT('',(-10.,50.,0.));
#15626=CARTESIAN_POINT('Origin',(15.,6.,0.));
#15627=CARTESIAN_POINT('',(-15.,6.,0.));
#15628=CARTESIAN_POINT('',(15.,6.,0.));
#15629=CARTESIAN_POINT('',(-15.,6.,0.));
#15630=CARTESIAN_POINT('Origin',(0.,0.,0.));
#15631=CARTESIAN_POINT('',(15.,6.,0.));
#15632=CARTESIAN_POINT('',(15.,6.,0.));
#15633=CARTESIAN_POINT('',(15.,-6.,0.));
#15634=CARTESIAN_POINT('Origin',(15.,0.,0.));
#15635=CARTESIAN_POINT('',(5.29150262212918,-6.,0.));
#15636=CARTESIAN_POINT('',(-15.,-6.,0.));
#15637=CARTESIAN_POINT('',(-5.29150262212918,-6.,0.));
#15638=CARTESIAN_POINT('Origin',(0.,0.,0.));
#15639=CARTESIAN_POINT('',(-15.,-6.,0.));
#15640=CARTESIAN_POINT('',(-15.,-6.,0.));
#15641=CARTESIAN_POINT('Origin',(-15.,0.,0.));
#15642=CARTESIAN_POINT('Origin',(0.,0.,0.));
#15643=CARTESIAN_POINT('',(5.29150262212918,-6.,0.));
#15644=CARTESIAN_POINT('',(-5.29150262212918,-6.,0.));
#15645=CARTESIAN_POINT('Origin',(15.,6.,0.));
#15646=CARTESIAN_POINT('',(15.,6.,0.));
#15647=CARTESIAN_POINT('Origin',(-15.,-6.,0.));
#15648=CARTESIAN_POINT('',(-15.,-6.,0.));
#15649=CARTESIAN_POINT('Origin',(15.,0.,0.));
#15650=CARTESIAN_POINT('',(15.,-6.,0.));
#15651=CARTESIAN_POINT('Origin',(-15.,-6.,0.));
#15652=CARTESIAN_POINT('Origin',(-15.,0.,0.));
#19825=UNCERTAINTY_MEASURE_WITH_UNIT(LENGTH_MEASURE(0.01),#19864,
'DISTANCE_ACCURACY_VALUE',
'Maximum model space distance between geometric entities at asserted c
onnectivities');
#19842=UNCERTAINTY_MEASURE_WITH_UNIT(LENGTH_MEASURE(0.01),#19864,
'DISTANCE_ACCURACY_VALUE',
'Maximum model space distance between geometric entities at asserted c
onnectivities');
#19846=(
GEOMETRIC_REPRESENTATION_CONTEXT(3)
GLOBAL_UNCERTAINTY_ASSIGNED_CONTEXT((#19825))
GLOBAL_UNIT_ASSIGNED_CONTEXT((#19864,#19866,#19867))
REPRESENTATION_CONTEXT('','3D')
);
#19863=(
GEOMETRIC_REPRESENTATION_CONTEXT(3)
GLOBAL_UNCERTAINTY_ASSIGNED_CONTEXT((#19842))
GLOBAL_UNIT_ASSIGNED_CONTEXT((#19864,#19866,#19867))
REPRESENTATION_CONTEXT('','3D')
);
#19864=(
LENGTH_UNIT()
NAMED_UNIT(*)
SI_UNIT(.MILLI.,.METRE.)
);
#19866=(
NAMED_UNIT(*)
PLANE_ANGLE_UNIT()
SI_UNIT($,.RADIAN.)
);
#19867=(
NAMED_UNIT(*)
SI_UNIT($,.STERADIAN.)
SOLID_ANGLE_UNIT()
);
#19871=SHAPE_DEFINITION_REPRESENTATION(#19891,#19937);
#19891=PRODUCT_DEFINITION_SHAPE('',$,#19958);
#19937=SHAPE_REPRESENTATION('',(#6827),#19846);
#19954=PRODUCT_DEFINITION_CONTEXT('part definition',#20016,'design');
#19958=PRODUCT_DEFINITION('Operating rocker','Operating rocker',#19978,
#19954);
#19978=PRODUCT_DEFINITION_FORMATION('',$,#20021);
#20016=APPLICATION_CONTEXT(
'Core Data for Automotive Mechanical Design Process');
#20017=PRODUCT_CONTEXT('part definition',#20016,'mechanical');
#20021=PRODUCT('Operating rocker','Operating rocker',$,(#20017));
#20039=PRESENTATION_STYLE_ASSIGNMENT((#20046));
#20046=SURFACE_STYLE_USAGE(.BOTH.,#20053);
#20053=SURFACE_SIDE_STYLE('',(#20060));
#20060=SURFACE_STYLE_FILL_AREA(#20067);
#20067=FILL_AREA_STYLE('Dark blue',(#20074));
#20074=FILL_AREA_STYLE_COLOUR('Dark blue',#20081);
#20081=COLOUR_RGB('Dark blue',0.0901960784313725,0.270588235294118,0.513725490196078);
ENDSEC;
END-ISO-10303-21;
